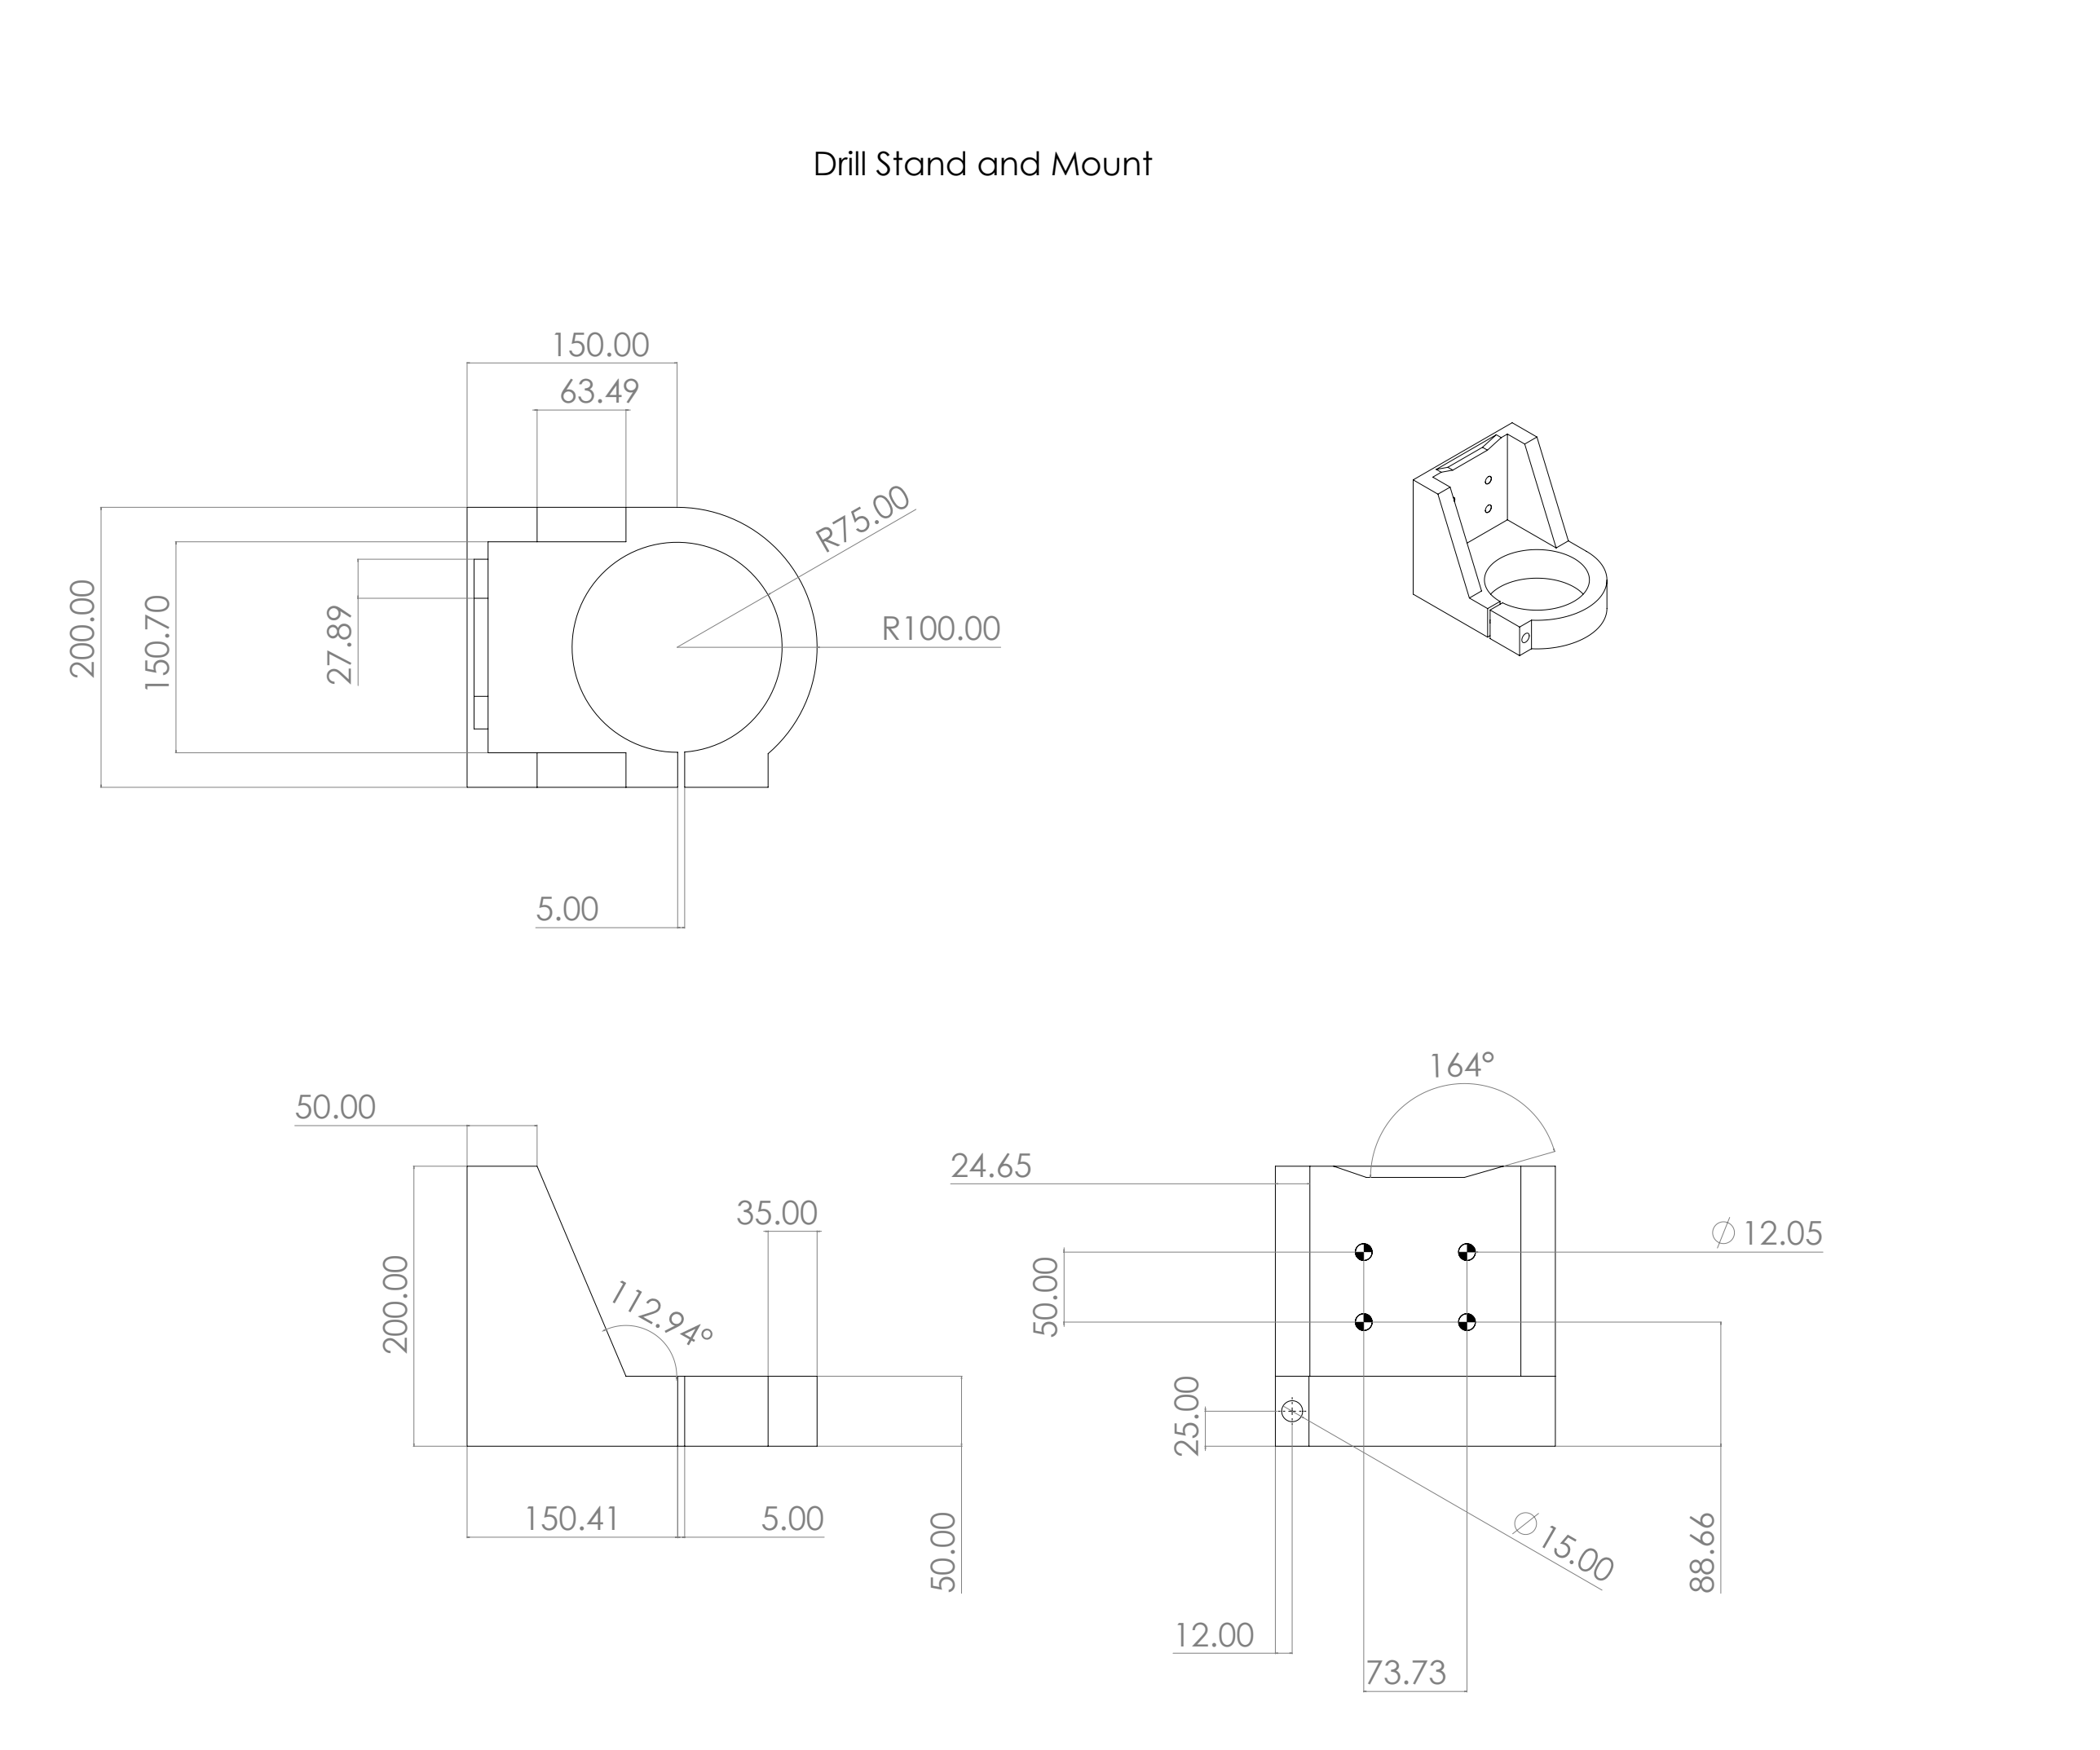
ISO-10303-21;
HEADER;
FILE_DESCRIPTION (('STEP AP214'),
    '1' );
FILE_NAME ('Drill Stand and Mount.step',
    '2026-10-24T00:09:50',
    ( '' ),
    ( '' ),
    'SwSTEP 2.0',
    'SolidWorks 2025',
    '' );
FILE_SCHEMA (( 'AUTOMOTIVE_DESIGN' ));
ENDSEC;

DATA;
#2=CARTESIAN_POINT ( 'NONE',  ( 367.9108539694884144, 44.41075299063183479, 74.99887465166234790 ) ) ;
#16=ORIENTED_EDGE ( 'NONE', *, *, #12011, .T. ) ;
#32=DIRECTION ( 'NONE',  ( 0.000000000000000000, 1.387778780781445182E-16, -1.000000000000000000 ) ) ;
#53=AXIS2_PLACEMENT_3D ( 'NONE', #26136, #19391, #25708 ) ;
#74=DIRECTION ( 'NONE',  ( 1.000000000000000000, -0.000000000000000000, -0.000000000000000000 ) ) ;
#117=VECTOR ( 'NONE', #24571, 1000.000000000000114 ) ;
#119=CIRCLE ( 'NONE', #12970, 75.00000000000002842 ) ;
#146=ORIENTED_EDGE ( 'NONE', *, *, #9436, .T. ) ;
#198=DIRECTION ( 'NONE',  ( 0.000000000000000000, 0.000000000000000000, -1.000000000000000000 ) ) ;
#214=CARTESIAN_POINT ( 'NONE',  ( 232.4999999999996305, 133.0668745871126930, 36.86484227207694886 ) ) ;
#251=CARTESIAN_POINT ( 'NONE',  ( 432.4999999999996589, 44.41075299063184190, 75.99342076785332267 ) ) ;
#260=CARTESIAN_POINT ( 'NONE',  ( 367.9108539694884144, 19.41075299063184900, 87.99671038392668265 ) ) ;
#262=DIRECTION ( 'NONE',  ( -0.000000000000000000, -1.024644424698391667E-16, 1.000000000000000000 ) ) ;
#272=DIRECTION ( 'NONE',  ( 0.000000000000000000, 0.000000000000000000, -1.000000000000000000 ) ) ;
#274=PRODUCT_DEFINITION_CONTEXT ( 'detailed design', #21209, 'design' ) ;
#283=LINE ( 'NONE', #20091, #23680 ) ;
#368=ORIENTED_EDGE ( 'NONE', *, *, #18128, .T. ) ;
#381=CARTESIAN_POINT ( 'NONE',  ( 502.4999999999996021, 44.41075299063184190, 75.35061095560295996 ) ) ;
#396=CARTESIAN_POINT ( 'NONE',  ( 232.4999999999996305, 494.4107529906318632, 75.35061095560301681 ) ) ;
#399=ORIENTED_EDGE ( 'NONE', *, *, #10312, .F. ) ;
#403=CARTESIAN_POINT ( 'NONE',  ( 232.4999999999996305, 494.4107529906318632, -75.35061095560287470 ) ) ;
#431=AXIS2_PLACEMENT_3D ( 'NONE', #7930, #14686, #18707 ) ;
#463=CARTESIAN_POINT ( 'NONE',  ( 267.4999999999996021, 194.4107529906317779, -100.0000000000000000 ) ) ;
#469=LINE ( 'NONE', #26317, #19493 ) ;
#496=DIRECTION ( 'NONE',  ( 0.000000000000000000, -1.000000000000000000, -1.214306433183764966E-16 ) ) ;
#499=DIRECTION ( 'NONE',  ( 0.000000000000000000, 0.000000000000000000, -1.000000000000000000 ) ) ;
#506=VERTEX_POINT ( 'NONE', #21563 ) ;
#545=ORIENTED_EDGE ( 'NONE', *, *, #17891, .F. ) ;
#558=VECTOR ( 'NONE', #22339, 1000.000000000000000 ) ;
#573=CARTESIAN_POINT ( 'NONE',  ( 232.4999999999996305, 44.41075299063184190, 75.35061095560295996 ) ) ;
#598=CIRCLE ( 'NONE', #1034, 7.499999999999992895 ) ;
#629=ORIENTED_EDGE ( 'NONE', *, *, #2343, .F. ) ;
#638=ADVANCED_FACE ( 'NONE', ( #4745 ), #27027, .F. ) ;
#722=ORIENTED_EDGE ( 'NONE', *, *, #6037, .F. ) ;
#743=EDGE_CURVE ( 'NONE', #20178, #23548, #16499, .T. ) ;
#762=ORIENTED_EDGE ( 'NONE', *, *, #3865, .T. ) ;
#776=CARTESIAN_POINT ( 'NONE',  ( 232.4999999999996305, 83.06687458711267880, 42.88984227207694033 ) ) ;
#797=DIRECTION ( 'NONE',  ( 0.000000000000000000, -1.000000000000000000, -1.214306433183764966E-16 ) ) ;
#819=LINE ( 'NONE', #9862, #20338 ) ;
#862=ADVANCED_FACE ( 'NONE', ( #20968 ), #22849, .F. ) ;
#863=VECTOR ( 'NONE', #10211, 1000.000000000000000 ) ;
#913=DIRECTION ( 'NONE',  ( 0.7071067811867438602, 8.659560562352529298E-17, 0.7071067811863512853 ) ) ;
#915=EDGE_LOOP ( 'NONE', ( #27754, #21554, #14846, #21946, #26433, #23940, #8844, #5653, #4028, #10467, #1807, #20190 ) ) ;
#967=ORIENTED_EDGE ( 'NONE', *, *, #14592, .T. ) ;
#1034=AXIS2_PLACEMENT_3D ( 'NONE', #27642, #24944, #3377 ) ;
#1059=AXIS2_PLACEMENT_3D ( 'NONE', #4720, #7463, #22546 ) ;
#1064=EDGE_CURVE ( 'NONE', #27217, #21245, #19801, .T. ) ;
#1075=ORIENTED_EDGE ( 'NONE', *, *, #26791, .T. ) ;
#1077=EDGE_LOOP ( 'NONE', ( #8320, #5448, #967, #19763 ) ) ;
#1096=EDGE_CURVE ( 'NONE', #27590, #27147, #25666, .T. ) ;
#1122=DIRECTION ( 'NONE',  ( -1.000000000000000000, 0.000000000000000000, -9.251858538542972814E-17 ) ) ;
#1154=CIRCLE ( 'NONE', #8503, 7.499999999999992895 ) ;
#1167=ORIENTED_EDGE ( 'NONE', *, *, #1977, .F. ) ;
#1168=AXIS2_PLACEMENT_3D ( 'NONE', #14174, #20345, #22928 ) ;
#1171=CARTESIAN_POINT ( 'NONE',  ( 432.4999999999996589, 19.41075299063184900, 95.49671038392668265 ) ) ;
#1182=EDGE_LOOP ( 'NONE', ( #21901, #2724, #8353, #8644 ) ) ;
#1229=DIRECTION ( 'NONE',  ( 0.000000000000000000, 0.000000000000000000, -1.000000000000000000 ) ) ;
#1251=ORIENTED_EDGE ( 'NONE', *, *, #28136, .T. ) ;
#1273=ORIENTED_EDGE ( 'NONE', *, *, #15927, .F. ) ;
#1283=DIRECTION ( 'NONE',  ( -1.000000000000000000, 0.000000000000000000, -0.000000000000000000 ) ) ;
#1360=EDGE_CURVE ( 'NONE', #5793, #19624, #20048, .T. ) ;
#1366=LINE ( 'NONE', #1775, #8493 ) ;
#1417=ORIENTED_EDGE ( 'NONE', *, *, #15927, .T. ) ;
#1464=MECHANICAL_DESIGN_GEOMETRIC_PRESENTATION_REPRESENTATION('',(#27159),#20745);
#1475=CARTESIAN_POINT ( 'NONE',  ( 282.4999999999996589, 19.41075299063184900, 87.99671038392668265 ) ) ;
#1484=DIRECTION ( 'NONE',  ( 0.000000000000000000, 1.214306433183764720E-16, -1.000000000000000000 ) ) ;
#1522=VECTOR ( 'NONE', #12404, 1000.000000000000000 ) ;
#1529=VECTOR ( 'NONE', #5297, 1000.000000000000000 ) ;
#1542=CARTESIAN_POINT ( 'NONE',  ( 232.4999999999996305, 133.0668745871126930, -30.83984227207694317 ) ) ;
#1550=VECTOR ( 'NONE', #20732, 1000.000000000000000 ) ;
#1571=EDGE_CURVE ( 'NONE', #11251, #16161, #1366, .T. ) ;
#1579=FACE_OUTER_BOUND ( 'NONE', #10470, .T. ) ;
#1613=PLANE ( 'NONE',  #28005 ) ;
#1630=DIRECTION ( 'NONE',  ( 0.000000000000000000, 0.000000000000000000, -1.000000000000000000 ) ) ;
#1644=DIRECTION ( 'NONE',  ( 0.000000000000000000, 0.000000000000000000, -1.000000000000000000 ) ) ;
#1696=ADVANCED_FACE ( 'NONE', ( #27494 ), #7832, .T. ) ;
#1734=FACE_OUTER_BOUND ( 'NONE', #4940, .T. ) ;
#1739=CARTESIAN_POINT ( 'NONE',  ( 232.4749999999995964, 83.06687458711267880, 36.86484227207694175 ) ) ;
#1775=CARTESIAN_POINT ( 'NONE',  ( 232.4999999999996305, 83.06687458711267880, 30.86484227207694886 ) ) ;
#1790=AXIS2_PLACEMENT_3D ( 'NONE', #5010, #4866, #7323 ) ;
#1794=CARTESIAN_POINT ( 'NONE',  ( 222.4999999999996021, 186.4134324495536248, 35.02193266779035952 ) ) ;
#1807=ORIENTED_EDGE ( 'NONE', *, *, #20147, .F. ) ;
#1840=ORIENTED_EDGE ( 'NONE', *, *, #2826, .T. ) ;
#1872=DIRECTION ( 'NONE',  ( 0.000000000000000000, -0.9458112779747414045, 0.3247168404252948615 ) ) ;
#1923=VECTOR ( 'NONE', #18549, 999.9999999999998863 ) ;
#1929=PRODUCT_DEFINITION_FORMATION_WITH_SPECIFIED_SOURCE ( 'ANY', '', #18972, .NOT_KNOWN. ) ;
#1977=EDGE_CURVE ( 'NONE', #23487, #10355, #2919, .T. ) ;
#1990=VECTOR ( 'NONE', #24485, 1000.000000000000000 ) ;
#2018=VERTEX_POINT ( 'NONE', #18010 ) ;
#2020=EDGE_LOOP ( 'NONE', ( #722, #7286, #1075, #6184, #18708, #10466 ) ) ;
#2033=CARTESIAN_POINT ( 'NONE',  ( 232.4999999999996305, 133.0668745871126930, 36.86484227207694886 ) ) ;
#2059=DIRECTION ( 'NONE',  ( 1.000000000000000000, -0.000000000000000000, -0.000000000000000000 ) ) ;
#2080=( NAMED_UNIT ( * ) PLANE_ANGLE_UNIT ( ) SI_UNIT ( $, .RADIAN. ) );
#2084=ORIENTED_EDGE ( 'NONE', *, *, #19529, .F. ) ;
#2085=ADVANCED_FACE ( 'NONE', ( #3611 ), #17365, .F. ) ;
#2130=DIRECTION ( 'NONE',  ( -1.000000000000000000, 0.000000000000000000, -9.251858538542972814E-17 ) ) ;
#2173=DIRECTION ( 'NONE',  ( 1.000000000000000000, -0.000000000000000000, -0.000000000000000000 ) ) ;
#2181=ORIENTED_EDGE ( 'NONE', *, *, #6541, .F. ) ;
#2210=DIRECTION ( 'NONE',  ( 1.000000000000000000, -0.000000000000000000, -0.000000000000000000 ) ) ;
#2216=AXIS2_PLACEMENT_3D ( 'NONE', #2525, #13468, #11754 ) ;
#2227=VERTEX_POINT ( 'NONE', #19949 ) ;
#2269=LINE ( 'NONE', #6873, #2943 ) ;
#2276=LINE ( 'NONE', #21684, #19032 ) ;
#2299=CARTESIAN_POINT ( 'NONE',  ( 232.4999999999996305, 133.0668745871126930, 36.86484227207694886 ) ) ;
#2316=CIRCLE ( 'NONE', #4166, 6.025000000000002132 ) ;
#2320=DIRECTION ( 'NONE',  ( 0.000000000000000000, 0.000000000000000000, 1.000000000000000000 ) ) ;
#2332=ORIENTED_EDGE ( 'NONE', *, *, #13602, .F. ) ;
#2343=EDGE_CURVE ( 'NONE', #9011, #23606, #20659, .T. ) ;
#2431=FACE_OUTER_BOUND ( 'NONE', #26216, .T. ) ;
#2438=CARTESIAN_POINT ( 'NONE',  ( 502.4999999999996021, 494.4107529906318632, -75.35061095560287470 ) ) ;
#2465=ORIENTED_EDGE ( 'NONE', *, *, #10551, .T. ) ;
#2484=DIRECTION ( 'NONE',  ( 0.000000000000000000, 1.272130549049657961E-16, -1.000000000000000000 ) ) ;
#2495=CARTESIAN_POINT ( 'NONE',  ( 232.4999999999996305, 83.06687458711267880, 36.86484227207694175 ) ) ;
#2525=CARTESIAN_POINT ( 'NONE',  ( 367.4999999999996021, -5.589247009368149222, 1.243177022048955014E-14 ) ) ;
#2543=AXIS2_PLACEMENT_3D ( 'NONE', #15014, #19732, #24191 ) ;
#2563=DIRECTION ( 'NONE',  ( 0.000000000000000000, 0.000000000000000000, -1.000000000000000000 ) ) ;
#2642=ORIENTED_EDGE ( 'NONE', *, *, #7765, .T. ) ;
#2649=CARTESIAN_POINT ( 'NONE',  ( 217.4999999999996305, 83.06687458711267880, 42.86484227207692754 ) ) ;
#2657=DIRECTION ( 'NONE',  ( 1.000000000000000000, -0.000000000000000000, -0.000000000000000000 ) ) ;
#2688=EDGE_CURVE ( 'NONE', #12924, #9277, #25082, .T. ) ;
#2697=LINE ( 'NONE', #24831, #15278 ) ;
#2699=AXIS2_PLACEMENT_3D ( 'NONE', #5745, #23135, #25425 ) ;
#2701=EDGE_CURVE ( 'NONE', #26144, #23757, #7603, .T. ) ;
#2717=DIRECTION ( 'NONE',  ( -0.000000000000000000, 0.000000000000000000, 1.000000000000000000 ) ) ;
#2724=ORIENTED_EDGE ( 'NONE', *, *, #25952, .F. ) ;
#2739=DIRECTION ( 'NONE',  ( 0.000000000000000000, 0.000000000000000000, -1.000000000000000000 ) ) ;
#2748=PLANE ( 'NONE',  #7343 ) ;
#2783=EDGE_LOOP ( 'NONE', ( #4645, #20293, #6997, #15217 ) ) ;
#2825=EDGE_LOOP ( 'NONE', ( #22493, #14150, #12355, #13881 ) ) ;
#2826=EDGE_CURVE ( 'NONE', #8811, #11251, #24124, .T. ) ;
#2868=ORIENTED_EDGE ( 'NONE', *, *, #7063, .T. ) ;
#2875=FACE_OUTER_BOUND ( 'NONE', #25974, .T. ) ;
#2876=AXIS2_PLACEMENT_3D ( 'NONE', #26536, #1872, #23869 ) ;
#2919=LINE ( 'NONE', #11703, #13120 ) ;
#2936=EDGE_CURVE ( 'NONE', #7575, #13442, #3014, .T. ) ;
#2943=VECTOR ( 'NONE', #15511, 1000.000000000000000 ) ;
#2944=CARTESIAN_POINT ( 'NONE',  ( 282.4999999999996589, 19.41075299063184900, 95.49671038392668265 ) ) ;
#2946=ORIENTED_EDGE ( 'NONE', *, *, #5275, .T. ) ;
#2947=AXIS2_PLACEMENT_3D ( 'NONE', #24170, #19708, #32 ) ;
#2977=VERTEX_POINT ( 'NONE', #17724 ) ;
#2983=CARTESIAN_POINT ( 'NONE',  ( 367.9108539694884144, 19.41075299063184900, 87.99671038392668265 ) ) ;
#3014=CIRCLE ( 'NONE', #9898, 75.00000000000002842 ) ;
#3017=CARTESIAN_POINT ( 'NONE',  ( 267.4999999999996021, 194.4107529906318064, 75.35061095560300259 ) ) ;
#3036=AXIS2_PLACEMENT_3D ( 'NONE', #20911, #5961, #12167 ) ;
#3045=DIRECTION ( 'NONE',  ( 0.000000000000000000, -0.000000000000000000, -1.000000000000000000 ) ) ;
#3065=CARTESIAN_POINT ( 'NONE',  ( 217.4999999999996305, 194.4107529906318064, -100.0000000000000000 ) ) ;
#3082=EDGE_LOOP ( 'NONE', ( #22866, #18073, #13925, #14229, #8531, #24826, #24828, #23547, #2946, #19715, #21670 ) ) ;
#3115=DIRECTION ( 'NONE',  ( 0.000000000000000000, 0.000000000000000000, 1.000000000000000000 ) ) ;
#3129=CARTESIAN_POINT ( 'NONE',  ( 330.9869376377542949, 44.41075299063183479, 288.0938197134494203 ) ) ;
#3165=DIRECTION ( 'NONE',  ( -1.000000000000000000, 0.000000000000000000, -0.000000000000000000 ) ) ;
#3199=ORIENTED_EDGE ( 'NONE', *, *, #28136, .F. ) ;
#3201=FACE_OUTER_BOUND ( 'NONE', #15790, .T. ) ;
#3215=CARTESIAN_POINT ( 'NONE',  ( 367.4999999999996021, 44.41075299063184900, 1.850330238640837654E-14 ) ) ;
#3216=ORIENTED_EDGE ( 'NONE', *, *, #8413, .T. ) ;
#3262=AXIS2_PLACEMENT_3D ( 'NONE', #21260, #14812, #17096 ) ;
#3268=DIRECTION ( 'NONE',  ( -0.000000000000000000, -0.000000000000000000, -1.000000000000000000 ) ) ;
#3274=ADVANCED_FACE ( 'NONE', ( #2875 ), #11668, .F. ) ;
#3284=AXIS2_PLACEMENT_3D ( 'NONE', #3500, #3782, #21026 ) ;
#3318=LINE ( 'NONE', #16414, #20270 ) ;
#3357=ORIENTED_EDGE ( 'NONE', *, *, #2688, .F. ) ;
#3363=ORIENTED_EDGE ( 'NONE', *, *, #15631, .T. ) ;
#3377=DIRECTION ( 'NONE',  ( 0.000000000000000000, 0.000000000000000000, -1.000000000000000000 ) ) ;
#3401=EDGE_CURVE ( 'NONE', #25274, #17486, #27497, .T. ) ;
#3414=LINE ( 'NONE', #3129, #3708 ) ;
#3427=ADVANCED_FACE ( 'NONE', ( #24692 ), #13792, .T. ) ;
#3443=PLANE ( 'NONE',  #2699 ) ;
#3473=CARTESIAN_POINT ( 'NONE',  ( 367.4999999999996021, -5.589247009368158103, 75.00000000000004263 ) ) ;
#3476=DIRECTION ( 'NONE',  ( -0.9209112846414913012, -0.3897722486529259789, 0.000000000000000000 ) ) ;
#3500=CARTESIAN_POINT ( 'NONE',  ( 217.4999999999996305, 44.41075299063186321, -100.0000000000000142 ) ) ;
#3549=EDGE_CURVE ( 'NONE', #18668, #22380, #28356, .T. ) ;
#3571=ORIENTED_EDGE ( 'NONE', *, *, #1096, .T. ) ;
#3611=FACE_OUTER_BOUND ( 'NONE', #25231, .T. ) ;
#3681=ORIENTED_EDGE ( 'NONE', *, *, #22426, .T. ) ;
#3708=VECTOR ( 'NONE', #3268, 1000.000000000000000 ) ;
#3782=DIRECTION ( 'NONE',  ( 0.000000000000000000, 1.214306433183764966E-16, -1.000000000000000000 ) ) ;
#3783=FACE_OUTER_BOUND ( 'NONE', #18224, .T. ) ;
#3787=DIRECTION ( 'NONE',  ( 0.000000000000000000, 0.000000000000000000, -1.000000000000000000 ) ) ;
#3799=CIRCLE ( 'NONE', #22158, 7.499999999999992895 ) ;
#3813=DIRECTION ( 'NONE',  ( 1.000000000000000000, -0.000000000000000000, -0.000000000000000000 ) ) ;
#3832=EDGE_CURVE ( 'NONE', #26471, #23612, #24621, .T. ) ;
#3849=ORIENTED_EDGE ( 'NONE', *, *, #22423, .T. ) ;
#3865=EDGE_CURVE ( 'NONE', #23487, #2018, #24718, .T. ) ;
#3909=FACE_OUTER_BOUND ( 'NONE', #1077, .T. ) ;
#3923=PLANE ( 'NONE',  #3284 ) ;
#3929=ORIENTED_EDGE ( 'NONE', *, *, #9136, .F. ) ;
#3942=ORIENTED_EDGE ( 'NONE', *, *, #20538, .T. ) ;
#3951=FACE_OUTER_BOUND ( 'NONE', #15568, .T. ) ;
#4026=AXIS2_PLACEMENT_3D ( 'NONE', #8368, #19568, #8512 ) ;
#4028=ORIENTED_EDGE ( 'NONE', *, *, #12389, .T. ) ;
#4056=CARTESIAN_POINT ( 'NONE',  ( 502.4999999999996021, 44.41075299063185611, -75.35061095560293154 ) ) ;
#4075=CARTESIAN_POINT ( 'NONE',  ( 232.4999999999996305, 133.0668745871126930, 36.86484227207694886 ) ) ;
#4078=DIRECTION ( 'NONE',  ( -0.000000000000000000, 0.2756732917354685064, -0.9612513907525602752 ) ) ;
#4084=CARTESIAN_POINT ( 'NONE',  ( 367.4999999999996021, 44.41075299063184900, 1.850330238640837654E-14 ) ) ;
#4105=EDGE_LOOP ( 'NONE', ( #25695, #5890, #24042, #26859 ) ) ;
#4130=ORIENTED_EDGE ( 'NONE', *, *, #8999, .F. ) ;
#4166=AXIS2_PLACEMENT_3D ( 'NONE', #13541, #19846, #5042 ) ;
#4176=VERTEX_POINT ( 'NONE', #18404 ) ;
#4263=DIRECTION ( 'NONE',  ( -0.000000000000000000, -0.000000000000000000, -1.000000000000000000 ) ) ;
#4266=CARTESIAN_POINT ( 'NONE',  ( 372.9108539694884144, -280.0000000000000568, 167.7200181511720132 ) ) ;
#4281=LINE ( 'NONE', #403, #10536 ) ;
#4286=ORIENTED_EDGE ( 'NONE', *, *, #7759, .F. ) ;
#4293=ADVANCED_FACE ( 'NONE', ( #21255, #14245, #12511, #7902, #16673 ), #3443, .T. ) ;
#4306=ORIENTED_EDGE ( 'NONE', *, *, #13602, .T. ) ;
#4325=FACE_OUTER_BOUND ( 'NONE', #11853, .T. ) ;
#4328=DIRECTION ( 'NONE',  ( 1.000000000000000000, -0.000000000000000000, -0.000000000000000000 ) ) ;
#4332=DIRECTION ( 'NONE',  ( 0.000000000000000000, 0.000000000000000000, -1.000000000000000000 ) ) ;
#4398=CARTESIAN_POINT ( 'NONE',  ( 217.4999999999996305, 133.0668745871126930, 42.86484227207692044 ) ) ;
#4430=DIRECTION ( 'NONE',  ( 0.000000000000000000, -1.000000000000000000, -1.214306433183764966E-16 ) ) ;
#4444=VECTOR ( 'NONE', #14125, 1000.000000000000000 ) ;
#4449=EDGE_LOOP ( 'NONE', ( #6153, #27694, #15526, #26157 ) ) ;
#4534=ADVANCED_FACE ( 'NONE', ( #11056 ), #19809, .F. ) ;
#4555=CARTESIAN_POINT ( 'NONE',  ( 367.9108539694884144, 44.41075299063183479, 167.7200181511720416 ) ) ;
#4563=CARTESIAN_POINT ( 'NONE',  ( 232.4749999999995964, 133.0668745871126930, 30.86484227207697018 ) ) ;
#4566=UNCERTAINTY_MEASURE_WITH_UNIT (LENGTH_MEASURE( 1.000000000000000082E-05 ), #22156, 'distance_accuracy_value', 'NONE');
#4567=CARTESIAN_POINT ( 'NONE',  ( 232.4999999999996305, 83.06687458711267880, 36.86484227207694175 ) ) ;
#4633=DIRECTION ( 'NONE',  ( 1.000000000000000000, 0.000000000000000000, 0.000000000000000000 ) ) ;
#4636=DIRECTION ( 'NONE',  ( 0.000000000000000000, 0.2756732917354685064, -0.9612513907525602752 ) ) ;
#4645=ORIENTED_EDGE ( 'NONE', *, *, #18540, .F. ) ;
#4675=CIRCLE ( 'NONE', #8361, 5.999999999999991118 ) ;
#4702=EDGE_CURVE ( 'NONE', #5949, #12519, #23528, .T. ) ;
#4708=ADVANCED_FACE ( 'NONE', ( #18520 ), #16434, .F. ) ;
#4720=CARTESIAN_POINT ( 'NONE',  ( 232.4999999999996305, 494.4107529906318632, 75.35061095560301681 ) ) ;
#4736=EDGE_CURVE ( 'NONE', #9830, #15470, #16371, .T. ) ;
#4745=FACE_OUTER_BOUND ( 'NONE', #22806, .T. ) ;
#4767=ORIENTED_EDGE ( 'NONE', *, *, #2701, .F. ) ;
#4788=DIRECTION ( 'NONE',  ( 0.000000000000000000, 1.214306433183764966E-16, -1.000000000000000000 ) ) ;
#4803=CARTESIAN_POINT ( 'NONE',  ( 222.4999999999996021, 186.4134324495536248, 35.02193266779035952 ) ) ;
#4810=ORIENTED_EDGE ( 'NONE', *, *, #10551, .F. ) ;
#4833=LINE ( 'NONE', #13913, #18573 ) ;
#4858=ADVANCED_FACE ( 'NONE', ( #6281, #19775 ), #15055, .F. ) ;
#4866=DIRECTION ( 'NONE',  ( 1.000000000000000000, -0.000000000000000000, -0.000000000000000000 ) ) ;
#4874=EDGE_CURVE ( 'NONE', #25738, #8109, #28102, .T. ) ;
#4940=EDGE_LOOP ( 'NONE', ( #13871, #12734, #13301, #11446 ) ) ;
#4980=EDGE_CURVE ( 'NONE', #22380, #7575, #6342, .T. ) ;
#4981=CARTESIAN_POINT ( 'NONE',  ( 217.4999999999996305, 194.4107529906318064, 100.0000000000000284 ) ) ;
#5010=CARTESIAN_POINT ( 'NONE',  ( 232.4999999999996305, 83.06687458711267880, -36.86484227207694175 ) ) ;
#5042=DIRECTION ( 'NONE',  ( 0.000000000000000000, 0.000000000000000000, -1.000000000000000000 ) ) ;
#5044=CARTESIAN_POINT ( 'NONE',  ( 217.4999999999996305, 83.06687458711267880, -36.86484227207694175 ) ) ;
#5045=ORIENTED_EDGE ( 'NONE', *, *, #6467, .F. ) ;
#5047=CARTESIAN_POINT ( 'NONE',  ( 367.4999999999996021, 44.41075299063184900, 1.850330238640837654E-14 ) ) ;
#5057=ADVANCED_BREP_SHAPE_REPRESENTATION ( '', ( #8800, #10637 ), #20272 ) ;
#5120=ORIENTED_EDGE ( 'NONE', *, *, #13622, .F. ) ;
#5156=AXIS2_PLACEMENT_3D ( 'NONE', #7372, #12115, #3045 ) ;
#5241=DIRECTION ( 'NONE',  ( 0.000000000000000000, 1.000000000000000000, 1.214306433183764966E-16 ) ) ;
#5261=AXIS2_PLACEMENT_3D ( 'NONE', #17632, #28252, #25824 ) ;
#5275=EDGE_CURVE ( 'NONE', #12260, #15470, #5914, .T. ) ;
#5297=DIRECTION ( 'NONE',  ( -1.000000000000000000, 0.000000000000000000, 0.000000000000000000 ) ) ;
#5306=ORIENTED_EDGE ( 'NONE', *, *, #17384, .T. ) ;
#5316=CARTESIAN_POINT ( 'NONE',  ( 232.4999999999996305, 83.06687458711267880, -36.86484227207694175 ) ) ;
#5339=CIRCLE ( 'NONE', #3036, 75.00000000000002842 ) ;
#5419=CARTESIAN_POINT ( 'NONE',  ( 282.4999999999996589, 19.41075299063184900, 80.49671038392669686 ) ) ;
#5448=ORIENTED_EDGE ( 'NONE', *, *, #15059, .F. ) ;
#5521=DIRECTION ( 'NONE',  ( 1.000000000000000000, -0.000000000000000000, -0.000000000000000000 ) ) ;
#5559=EDGE_CURVE ( 'NONE', #17744, #5793, #16676, .T. ) ;
#5587=CARTESIAN_POINT ( 'NONE',  ( 232.4999999999996305, 186.4134324495536248, -35.02193266779035952 ) ) ;
#5610=CARTESIAN_POINT ( 'NONE',  ( 222.4999999999996021, 0.000000000000000000, 0.000000000000000000 ) ) ;
#5614=DIRECTION ( 'NONE',  ( 1.000000000000000000, 0.000000000000000000, 0.000000000000000000 ) ) ;
#5627=AXIS2_PLACEMENT_3D ( 'NONE', #21043, #25363, #1229 ) ;
#5647=AXIS2_PLACEMENT_3D ( 'NONE', #2495, #2210, #11285 ) ;
#5653=ORIENTED_EDGE ( 'NONE', *, *, #14358, .F. ) ;
#5745=CARTESIAN_POINT ( 'NONE',  ( 217.4999999999996305, 44.41075299063183479, 100.0000000000000142 ) ) ;
#5767=ORIENTED_EDGE ( 'NONE', *, *, #6544, .F. ) ;
#5769=LINE ( 'NONE', #10231, #12506 ) ;
#5791=ORIENTED_EDGE ( 'NONE', *, *, #28135, .T. ) ;
#5793=VERTEX_POINT ( 'NONE', #573 ) ;
#5808=VERTEX_POINT ( 'NONE', #7467 ) ;
#5810=ORIENTED_EDGE ( 'NONE', *, *, #7765, .F. ) ;
#5834=DIRECTION ( 'NONE',  ( 1.000000000000000000, 0.000000000000000000, 0.000000000000000000 ) ) ;
#5859=ADVANCED_FACE ( 'NONE', ( #24704 ), #17949, .F. ) ;
#5890=ORIENTED_EDGE ( 'NONE', *, *, #10649, .T. ) ;
#5895=ORIENTED_EDGE ( 'NONE', *, *, #11648, .F. ) ;
#5897=ORIENTED_EDGE ( 'NONE', *, *, #21978, .T. ) ;
#5902=EDGE_LOOP ( 'NONE', ( #11688, #4767 ) ) ;
#5910=ORIENTED_EDGE ( 'NONE', *, *, #2936, .T. ) ;
#5911=FACE_OUTER_BOUND ( 'NONE', #4105, .T. ) ;
#5913=DIRECTION ( 'NONE',  ( 0.7071067811865474617, 8.659560562354932858E-17, 0.7071067811865474617 ) ) ;
#5914=CIRCLE ( 'NONE', #22432, 100.0000000000000284 ) ;
#5920=AXIS2_PLACEMENT_3D ( 'NONE', #2299, #8923, #15973 ) ;
#5925=CARTESIAN_POINT ( 'NONE',  ( 232.4999999999996305, 83.06687458711267880, 42.88984227207694033 ) ) ;
#5930=EDGE_LOOP ( 'NONE', ( #1167, #21949, #23539, #4306 ) ) ;
#5938=DIRECTION ( 'NONE',  ( 0.000000000000000000, -1.000000000000000000, -1.214306433183764966E-16 ) ) ;
#5946=CYLINDRICAL_SURFACE ( 'NONE', #20961, 7.499999999999992895 ) ;
#5949=VERTEX_POINT ( 'NONE', #8308 ) ;
#5957=AXIS2_PLACEMENT_3D ( 'NONE', #19610, #25787, #25928 ) ;
#5961=DIRECTION ( 'NONE',  ( 0.000000000000000000, -1.000000000000000000, -1.214306433183764966E-16 ) ) ;
#5981=APPLICATION_CONTEXT ( 'automotive_design' ) ;
#6024=CARTESIAN_POINT ( 'NONE',  ( 222.4999999999996021, 194.4107529906318064, -62.90796922943941638 ) ) ;
#6030=CARTESIAN_POINT ( 'NONE',  ( 232.4999999999996305, 44.41075299063184190, 75.35061095560295996 ) ) ;
#6037=EDGE_CURVE ( 'NONE', #9011, #27217, #14634, .T. ) ;
#6040=ORIENTED_EDGE ( 'NONE', *, *, #12231, .T. ) ;
#6047=EDGE_LOOP ( 'NONE', ( #16873, #9356, #10053, #17070 ) ) ;
#6050=AXIS2_PLACEMENT_3D ( 'NONE', #1475, #23178, #14851 ) ;
#6054=CARTESIAN_POINT ( 'NONE',  ( 232.4749999999995964, 133.0668745871126930, 42.86484227207692044 ) ) ;
#6091=CARTESIAN_POINT ( 'NONE',  ( 222.4999999999996021, 186.4134324495536248, -35.02193266779035952 ) ) ;
#6102=ORIENTED_EDGE ( 'NONE', *, *, #5275, .F. ) ;
#6117=CARTESIAN_POINT ( 'NONE',  ( 372.9108539694884144, 44.41075299063183479, 74.80456309157131045 ) ) ;
#6118=EDGE_LOOP ( 'NONE', ( #7668, #22373, #5910, #21610 ) ) ;
#6145=FACE_OUTER_BOUND ( 'NONE', #19193, .T. ) ;
#6153=ORIENTED_EDGE ( 'NONE', *, *, #28236, .F. ) ;
#6184=ORIENTED_EDGE ( 'NONE', *, *, #14358, .T. ) ;
#6191=VECTOR ( 'NONE', #14804, 1000.000000000000000 ) ;
#6229=ORIENTED_EDGE ( 'NONE', *, *, #14714, .F. ) ;
#6280=CARTESIAN_POINT ( 'NONE',  ( 367.9108539694884144, -5.589247009368157215, 74.99887465166234790 ) ) ;
#6281=FACE_BOUND ( 'NONE', #16596, .T. ) ;
#6290=DIRECTION ( 'NONE',  ( 0.000000000000000000, -1.000000000000000000, -1.214306433183764966E-16 ) ) ;
#6294=EDGE_CURVE ( 'NONE', #8492, #5793, #20064, .T. ) ;
#6322=VECTOR ( 'NONE', #27537, 1000.000000000000000 ) ;
#6342=CIRCLE ( 'NONE', #2216, 75.00000000000002842 ) ;
#6346=CARTESIAN_POINT ( 'NONE',  ( 367.9108539694884144, -280.0000000000000568, 167.7200181511720132 ) ) ;
#6443=ORIENTED_EDGE ( 'NONE', *, *, #6541, .T. ) ;
#6467=EDGE_CURVE ( 'NONE', #9950, #15333, #14681, .T. ) ;
#6481=ORIENTED_EDGE ( 'NONE', *, *, #27821, .F. ) ;
#6492=LINE ( 'NONE', #14988, #17920 ) ;
#6541=EDGE_CURVE ( 'NONE', #2227, #12260, #17591, .T. ) ;
#6544=EDGE_CURVE ( 'NONE', #9950, #20572, #21908, .T. ) ;
#6591=UNCERTAINTY_MEASURE_WITH_UNIT (LENGTH_MEASURE( 1.000000000000000082E-05 ), #17884, 'distance_accuracy_value', 'NONE');
#6635=CARTESIAN_POINT ( 'NONE',  ( 217.4999999999996305, 194.4107529906318064, -75.35061095560291733 ) ) ;
#6642=DIRECTION ( 'NONE',  ( -0.000000000000000000, -0.000000000000000000, -1.000000000000000000 ) ) ;
#6652=CARTESIAN_POINT ( 'NONE',  ( 232.4999999999996305, 133.0668745871126930, -30.83984227207694317 ) ) ;
#6673=CARTESIAN_POINT ( 'NONE',  ( 222.4999999999996021, 186.4134324495536248, -35.02193266779035952 ) ) ;
#6686=ORIENTED_EDGE ( 'NONE', *, *, #15833, .F. ) ;
#6706=ORIENTED_EDGE ( 'NONE', *, *, #11340, .F. ) ;
#6733=DIRECTION ( 'NONE',  ( 1.000000000000000000, 0.000000000000000000, 0.000000000000000000 ) ) ;
#6738=DIRECTION ( 'NONE',  ( 0.000000000000000000, 1.000000000000000000, 1.214306433183764966E-16 ) ) ;
#6742=CIRCLE ( 'NONE', #20511, 5.999999999999977796 ) ;
#6777=DIRECTION ( 'NONE',  ( 1.000000000000000000, 0.000000000000000000, 0.000000000000000000 ) ) ;
#6803=DIRECTION ( 'NONE',  ( 0.000000000000000000, 1.387778780781445182E-16, -1.000000000000000000 ) ) ;
#6873=CARTESIAN_POINT ( 'NONE',  ( 232.4999999999996305, 194.4107529906318064, 288.0938197134494203 ) ) ;
#6888=EDGE_LOOP ( 'NONE', ( #24221, #12671, #19443, #20155 ) ) ;
#6894=EDGE_LOOP ( 'NONE', ( #10162, #3199, #25412, #6040 ) ) ;
#6941=EDGE_CURVE ( 'NONE', #13442, #25647, #10676, .T. ) ;
#6949=DIRECTION ( 'NONE',  ( 1.000000000000000000, 0.000000000000000000, 0.000000000000000000 ) ) ;
#6959=LINE ( 'NONE', #4803, #558 ) ;
#6969=EDGE_LOOP ( 'NONE', ( #17569, #7993 ) ) ;
#6997=ORIENTED_EDGE ( 'NONE', *, *, #22454, .T. ) ;
#7026=VECTOR ( 'NONE', #15775, 1000.000000000000000 ) ;
#7046=CARTESIAN_POINT ( 'NONE',  ( 232.4999999999996305, 83.06687458711267880, -30.83984227207693607 ) ) ;
#7063=EDGE_CURVE ( 'NONE', #17486, #25274, #22035, .T. ) ;
#7076=EDGE_CURVE ( 'NONE', #26636, #22380, #12512, .T. ) ;
#7149=DIRECTION ( 'NONE',  ( -1.000000000000000000, 0.000000000000000000, -0.000000000000000000 ) ) ;
#7154=VERTEX_POINT ( 'NONE', #10481 ) ;
#7190=VECTOR ( 'NONE', #19587, 1000.000000000000114 ) ;
#7224=CARTESIAN_POINT ( 'NONE',  ( 232.4999999999996305, 133.0668745871126930, -42.88984227207694744 ) ) ;
#7237=DIRECTION ( 'NONE',  ( 1.000000000000000000, -0.000000000000000000, -0.000000000000000000 ) ) ;
#7250=DIRECTION ( 'NONE',  ( 1.000000000000000000, -0.000000000000000000, -0.000000000000000000 ) ) ;
#7276=ADVANCED_FACE ( 'NONE', ( #15205 ), #15490, .F. ) ;
#7277=CARTESIAN_POINT ( 'NONE',  ( 232.4999999999996305, 44.41075299063185611, -75.35061095560293154 ) ) ;
#7286=ORIENTED_EDGE ( 'NONE', *, *, #2343, .T. ) ;
#7290=AXIS2_PLACEMENT_3D ( 'NONE', #16778, #7870, #22824 ) ;
#7295=ORIENTED_EDGE ( 'NONE', *, *, #8807, .T. ) ;
#7323=DIRECTION ( 'NONE',  ( 0.000000000000000000, 0.000000000000000000, -1.000000000000000000 ) ) ;
#7343=AXIS2_PLACEMENT_3D ( 'NONE', #22586, #15989, #7502 ) ;
#7372=CARTESIAN_POINT ( 'NONE',  ( 217.4999999999996305, 194.4107529906318064, 288.0938197134494203 ) ) ;
#7405=CIRCLE ( 'NONE', #24832, 6.025000000000002132 ) ;
#7410=DIRECTION ( 'NONE',  ( 0.000000000000000000, 0.000000000000000000, -1.000000000000000000 ) ) ;
#7435=CARTESIAN_POINT ( 'NONE',  ( 232.4999999999996305, 194.4107529906318064, 75.35061095560297417 ) ) ;
#7440=EDGE_CURVE ( 'NONE', #2977, #7154, #20209, .T. ) ;
#7463=DIRECTION ( 'NONE',  ( 1.000000000000000000, 0.000000000000000000, 0.000000000000000000 ) ) ;
#7467=CARTESIAN_POINT ( 'NONE',  ( 217.4999999999996305, -5.589247009368136787, -100.0000000000000142 ) ) ;
#7480=VERTEX_POINT ( 'NONE', #5925 ) ;
#7484=VECTOR ( 'NONE', #18367, 1000.000000000000000 ) ;
#7488=CARTESIAN_POINT ( 'NONE',  ( 232.4999999999996305, 83.06687458711267880, 36.86484227207694175 ) ) ;
#7496=CARTESIAN_POINT ( 'NONE',  ( 222.4999999999996021, 186.4134324495536248, -35.02193266779035952 ) ) ;
#7502=DIRECTION ( 'NONE',  ( 0.3897722486529259234, -0.9209112846414911902, 0.000000000000000000 ) ) ;
#7504=DIRECTION ( 'NONE',  ( 0.000000000000000000, -1.000000000000000000, -1.214306433183764966E-16 ) ) ;
#7516=CARTESIAN_POINT ( 'NONE',  ( 222.4999999999996021, 194.4107529906318064, -62.90796922943941638 ) ) ;
#7537=CARTESIAN_POINT ( 'NONE',  ( 222.4999999999996021, 194.4107529906318064, 58.31593845887894645 ) ) ;
#7543=LINE ( 'NONE', #25476, #19037 ) ;
#7553=ORIENTED_EDGE ( 'NONE', *, *, #1360, .T. ) ;
#7559=ADVANCED_FACE ( 'NONE', ( #23735 ), #19760, .F. ) ;
#7575=VERTEX_POINT ( 'NONE', #25740 ) ;
#7602=DIRECTION ( 'NONE',  ( 0.000000000000000000, 0.000000000000000000, -1.000000000000000000 ) ) ;
#7603=CIRCLE ( 'NONE', #1168, 6.025000000000002132 ) ;
#7619=AXIS2_PLACEMENT_3D ( 'NONE', #27597, #3476, #23984 ) ;
#7623=DIRECTION ( 'NONE',  ( -9.251858538542974046E-17, -1.214306433183764966E-16, 1.000000000000000000 ) ) ;
#7624=EDGE_CURVE ( 'NONE', #12356, #16763, #6492, .T. ) ;
#7632=ADVANCED_FACE ( 'NONE', ( #19284, #19571 ), #1613, .F. ) ;
#7641=EDGE_CURVE ( 'NONE', #23548, #20178, #2316, .T. ) ;
#7649=DIRECTION ( 'NONE',  ( 0.7071067811867438602, 0.000000000000000000, -0.7071067811863512853 ) ) ;
#7651=ORIENTED_EDGE ( 'NONE', *, *, #8934, .T. ) ;
#7668=ORIENTED_EDGE ( 'NONE', *, *, #8934, .F. ) ;
#7669=CARTESIAN_POINT ( 'NONE',  ( 432.4999999999996589, -5.589247009368158103, 75.99342076785332267 ) ) ;
#7685=CLOSED_SHELL ( 'NONE', ( #27662, #5859, #10923, #13213, #638, #25140, #12744, #862, #18950, #19519, #7276, #21054, #26875, #12538, #12366, #2085, #16790, #21383, #15295, #4293, #3427, #10099, #7950, #11235, #9891, #10487, #18643, #7632, #4858, #26174, #23715, #1696, #14081, #13988, #21540, #15788, #18376, #21415, #23268, #16251, #4534, #4708, #3274, #7559 ) ) ;
#7720=AXIS2_PLACEMENT_3D ( 'NONE', #4084, #10706, #6803 ) ;
#7759=EDGE_CURVE ( 'NONE', #27147, #23757, #27294, .T. ) ;
#7765=EDGE_CURVE ( 'NONE', #8109, #8669, #20694, .T. ) ;
#7775=DIRECTION ( 'NONE',  ( 0.000000000000000000, 0.000000000000000000, -1.000000000000000000 ) ) ;
#7812=AXIS2_PLACEMENT_3D ( 'NONE', #24129, #25985, #17652 ) ;
#7825=FACE_OUTER_BOUND ( 'NONE', #5930, .T. ) ;
#7827=VECTOR ( 'NONE', #4078, 1000.000000000000000 ) ;
#7832=PLANE ( 'NONE',  #11266 ) ;
#7865=EDGE_CURVE ( 'NONE', #23614, #17607, #12009, .T. ) ;
#7870=DIRECTION ( 'NONE',  ( 0.000000000000000000, -1.000000000000000000, -1.214306433183764966E-16 ) ) ;
#7885=ORIENTED_EDGE ( 'NONE', *, *, #6941, .T. ) ;
#7893=ORIENTED_EDGE ( 'NONE', *, *, #21439, .T. ) ;
#7902=FACE_BOUND ( 'NONE', #21379, .T. ) ;
#7908=CARTESIAN_POINT ( 'NONE',  ( 232.4999999999996305, 133.0668745871126930, 30.83984227207694317 ) ) ;
#7930=CARTESIAN_POINT ( 'NONE',  ( 232.4999999999996305, 83.06687458711267880, -36.86484227207694175 ) ) ;
#7950=ADVANCED_FACE ( 'NONE', ( #27995 ), #16818, .T. ) ;
#7952=ORIENTED_EDGE ( 'NONE', *, *, #28236, .T. ) ;
#7993=ORIENTED_EDGE ( 'NONE', *, *, #6467, .T. ) ;
#7996=CARTESIAN_POINT ( 'NONE',  ( 217.4999999999996305, 194.4107529906318064, 75.35061095560300259 ) ) ;
#8019=VERTEX_POINT ( 'NONE', #2 ) ;
#8036=CARTESIAN_POINT ( 'NONE',  ( 367.4999999999996021, 44.41075299063183479, 100.0000000000000284 ) ) ;
#8084=EDGE_LOOP ( 'NONE', ( #2332, #11399 ) ) ;
#8090=LINE ( 'NONE', #21435, #26330 ) ;
#8104=CARTESIAN_POINT ( 'NONE',  ( 232.4999999999996305, 133.0668745871126930, 36.86484227207694886 ) ) ;
#8109=VERTEX_POINT ( 'NONE', #21970 ) ;
#8145=EDGE_CURVE ( 'NONE', #25647, #8109, #11354, .T. ) ;
#8187=AXIS2_PLACEMENT_3D ( 'NONE', #5610, #20975, #14523 ) ;
#8196=VECTOR ( 'NONE', #11564, 1000.000000000000000 ) ;
#8223=AXIS2_PLACEMENT_3D ( 'NONE', #22103, #17647, #272 ) ;
#8249=ORIENTED_EDGE ( 'NONE', *, *, #16395, .F. ) ;
#8284=CARTESIAN_POINT ( 'NONE',  ( 432.4999999999996589, 44.41075299063184190, 100.0000000000000426 ) ) ;
#8308=CARTESIAN_POINT ( 'NONE',  ( 222.4999999999996021, 194.4107529906318064, -62.90796922943941638 ) ) ;
#8320=ORIENTED_EDGE ( 'NONE', *, *, #7076, .F. ) ;
#8353=ORIENTED_EDGE ( 'NONE', *, *, #7759, .T. ) ;
#8361=AXIS2_PLACEMENT_3D ( 'NONE', #13102, #28151, #19828 ) ;
#8368=CARTESIAN_POINT ( 'NONE',  ( 232.4749999999995964, 83.06687458711267880, 36.86484227207694175 ) ) ;
#8386=AXIS2_PLACEMENT_3D ( 'NONE', #22410, #9345, #10679 ) ;
#8413=EDGE_CURVE ( 'NONE', #14199, #12077, #26383, .T. ) ;
#8417=CARTESIAN_POINT ( 'NONE',  ( 232.4999999999996305, 133.0668745871126930, -36.86484227207694886 ) ) ;
#8446=CIRCLE ( 'NONE', #17152, 7.499999999999992895 ) ;
#8492=VERTEX_POINT ( 'NONE', #7435 ) ;
#8493=VECTOR ( 'NONE', #21460, 1000.000000000000000 ) ;
#8503=AXIS2_PLACEMENT_3D ( 'NONE', #26448, #6777, #20285 ) ;
#8504=CARTESIAN_POINT ( 'NONE',  ( 232.4999999999996305, 133.0668745871126930, 42.88984227207694744 ) ) ;
#8510=LINE ( 'NONE', #28304, #13371 ) ;
#8512=DIRECTION ( 'NONE',  ( 0.000000000000000000, 0.000000000000000000, -1.000000000000000000 ) ) ;
#8531=ORIENTED_EDGE ( 'NONE', *, *, #21543, .F. ) ;
#8544=VECTOR ( 'NONE', #15052, 1000.000000000000000 ) ;
#8554=DIRECTION ( 'NONE',  ( 0.000000000000000000, -1.000000000000000000, -1.214306433183764966E-16 ) ) ;
#8644=ORIENTED_EDGE ( 'NONE', *, *, #18445, .T. ) ;
#8655=CARTESIAN_POINT ( 'NONE',  ( 232.4999999999996305, 83.06687458711267880, -36.86484227207694175 ) ) ;
#8667=VECTOR ( 'NONE', #22291, 1000.000000000000000 ) ;
#8669=VERTEX_POINT ( 'NONE', #6117 ) ;
#8721=LINE ( 'NONE', #9005, #20015 ) ;
#8770=ORIENTED_EDGE ( 'NONE', *, *, #4874, .T. ) ;
#8782=AXIS2_PLACEMENT_3D ( 'NONE', #26095, #21226, #13054 ) ;
#8783=CYLINDRICAL_SURFACE ( 'NONE', #24513, 7.499999999999992895 ) ;
#8785=VECTOR ( 'NONE', #15600, 1000.000000000000000 ) ;
#8800=MANIFOLD_SOLID_BREP ( '\X2\00d8\X0\12.0mm Dowel Hole2[2]', #7685 ) ;
#8807=EDGE_CURVE ( 'NONE', #12519, #26013, #6959, .T. ) ;
#8811=VERTEX_POINT ( 'NONE', #2649 ) ;
#8844=ORIENTED_EDGE ( 'NONE', *, *, #14697, .F. ) ;
#8848=VECTOR ( 'NONE', #2717, 1000.000000000000000 ) ;
#8850=ORIENTED_EDGE ( 'NONE', *, *, #15590, .T. ) ;
#8923=DIRECTION ( 'NONE',  ( 1.000000000000000000, -0.000000000000000000, -0.000000000000000000 ) ) ;
#8934=EDGE_CURVE ( 'NONE', #23123, #8669, #119, .T. ) ;
#8953=CARTESIAN_POINT ( 'NONE',  ( 217.4999999999996305, -5.589247009368160768, 100.0000000000000142 ) ) ;
#8961=DIRECTION ( 'NONE',  ( 0.000000000000000000, -0.9612513907525602752, -0.2756732917354685064 ) ) ;
#8999=EDGE_CURVE ( 'NONE', #14199, #17744, #25339, .T. ) ;
#9005=CARTESIAN_POINT ( 'NONE',  ( 232.4999999999996305, 133.0668745871126930, -42.88984227207694744 ) ) ;
#9011=VERTEX_POINT ( 'NONE', #14571 ) ;
#9049=EDGE_LOOP ( 'NONE', ( #5045, #9127, #21873, #10647 ) ) ;
#9127=ORIENTED_EDGE ( 'NONE', *, *, #6544, .T. ) ;
#9128=CARTESIAN_POINT ( 'NONE',  ( 367.4999999999996021, 44.41075299063185611, -75.00000000000001421 ) ) ;
#9136=EDGE_CURVE ( 'NONE', #7154, #24450, #22600, .T. ) ;
#9188=PLANE ( 'NONE',  #1059 ) ;
#9239=LINE ( 'NONE', #7516, #4444 ) ;
#9245=VECTOR ( 'NONE', #74, 1000.000000000000000 ) ;
#9260=ORIENTED_EDGE ( 'NONE', *, *, #1977, .T. ) ;
#9277=VERTEX_POINT ( 'NONE', #5587 ) ;
#9340=CARTESIAN_POINT ( 'NONE',  ( 232.4999999999996305, 83.06687458711267880, -30.83984227207693607 ) ) ;
#9345=DIRECTION ( 'NONE',  ( 1.000000000000000000, -0.000000000000000000, -0.000000000000000000 ) ) ;
#9350=ORIENTED_EDGE ( 'NONE', *, *, #19705, .F. ) ;
#9351=AXIS2_PLACEMENT_3D ( 'NONE', #5047, #7504, #22587 ) ;
#9356=ORIENTED_EDGE ( 'NONE', *, *, #18501, .T. ) ;
#9432=VERTEX_POINT ( 'NONE', #4981 ) ;
#9436=EDGE_CURVE ( 'NONE', #20572, #21229, #3799, .T. ) ;
#9456=AXIS2_PLACEMENT_3D ( 'NONE', #8104, #5521, #1630 ) ;
#9522=ORIENTED_EDGE ( 'NONE', *, *, #27821, .T. ) ;
#9579=VECTOR ( 'NONE', #12937, 1000.000000000000000 ) ;
#9618=DIRECTION ( 'NONE',  ( 0.000000000000000000, 0.000000000000000000, -1.000000000000000000 ) ) ;
#9680=DIRECTION ( 'NONE',  ( 0.000000000000000000, 0.000000000000000000, -1.000000000000000000 ) ) ;
#9684=EDGE_LOOP ( 'NONE', ( #15667, #20286 ) ) ;
#9699=VECTOR ( 'NONE', #24842, 1000.000000000000000 ) ;
#9700=CARTESIAN_POINT ( 'NONE',  ( 502.4999999999996021, 494.4107529906318632, 75.35061095560301681 ) ) ;
#9716=EDGE_CURVE ( 'NONE', #8492, #26679, #21628, .T. ) ;
#9740=VERTEX_POINT ( 'NONE', #21201 ) ;
#9813=CIRCLE ( 'NONE', #14889, 6.025000000000002132 ) ;
#9830=VERTEX_POINT ( 'NONE', #13169 ) ;
#9862=CARTESIAN_POINT ( 'NONE',  ( 217.4999999999996305, 44.41075299063186321, -100.0000000000000142 ) ) ;
#9891=ADVANCED_FACE ( 'NONE', ( #24926 ), #16175, .T. ) ;
#9898=AXIS2_PLACEMENT_3D ( 'NONE', #13424, #11273, #2484 ) ;
#9950=VERTEX_POINT ( 'NONE', #2944 ) ;
#10053=ORIENTED_EDGE ( 'NONE', *, *, #19705, .T. ) ;
#10063=VECTOR ( 'NONE', #7250, 1000.000000000000000 ) ;
#10071=DIRECTION ( 'NONE',  ( 0.7071067811865474617, 0.000000000000000000, -0.7071067811865474617 ) ) ;
#10079=ORIENTED_EDGE ( 'NONE', *, *, #1360, .F. ) ;
#10086=EDGE_LOOP ( 'NONE', ( #7885, #14505, #2642, #13298 ) ) ;
#10099=ADVANCED_FACE ( 'NONE', ( #25755 ), #3923, .T. ) ;
#10127=CARTESIAN_POINT ( 'NONE',  ( 232.4999999999996305, 186.4134324495536248, 35.02193266779035952 ) ) ;
#10162=ORIENTED_EDGE ( 'NONE', *, *, #26141, .T. ) ;
#10197=PLANE ( 'NONE',  #27845 ) ;
#10211=DIRECTION ( 'NONE',  ( -0.000000000000000000, -9.208809080520486542E-17, 1.000000000000000000 ) ) ;
#10231=CARTESIAN_POINT ( 'NONE',  ( 432.4999999999996589, -5.589247009368160768, 100.0000000000000426 ) ) ;
#10241=VECTOR ( 'NONE', #5913, 1000.000000000000114 ) ;
#10248=DIRECTION ( 'NONE',  ( 1.000000000000000000, -0.000000000000000000, -0.000000000000000000 ) ) ;
#10258=DIRECTION ( 'NONE',  ( -1.000000000000000000, 0.000000000000000000, 0.000000000000000000 ) ) ;
#10312=EDGE_CURVE ( 'NONE', #16161, #19401, #3318, .T. ) ;
#10315=PLANE ( 'NONE',  #8782 ) ;
#10336=DIRECTION ( 'NONE',  ( 0.000000000000000000, -1.000000000000000000, -1.214306433183764966E-16 ) ) ;
#10341=CARTESIAN_POINT ( 'NONE',  ( 232.4999999999996305, 194.4107529906318064, -62.90796922943941638 ) ) ;
#10350=CARTESIAN_POINT ( 'NONE',  ( 372.9108539694884144, 19.41075299063184900, 87.99671038392668265 ) ) ;
#10355=VERTEX_POINT ( 'NONE', #1171 ) ;
#10357=ORIENTED_EDGE ( 'NONE', *, *, #8145, .F. ) ;
#10359=VECTOR ( 'NONE', #797, 1000.000000000000000 ) ;
#10367=EDGE_LOOP ( 'NONE', ( #1273, #1840, #27064, #8850 ) ) ;
#10369=DIRECTION ( 'NONE',  ( 1.000000000000000000, -0.000000000000000000, -0.000000000000000000 ) ) ;
#10384=DIRECTION ( 'NONE',  ( -1.000000000000000000, 0.000000000000000000, -0.000000000000000000 ) ) ;
#10415=CARTESIAN_POINT ( 'NONE',  ( 217.4999999999996305, 44.41075299063186321, -100.0000000000000142 ) ) ;
#10416=DIRECTION ( 'NONE',  ( 0.000000000000000000, 0.000000000000000000, 1.000000000000000000 ) ) ;
#10466=ORIENTED_EDGE ( 'NONE', *, *, #1064, .F. ) ;
#10467=ORIENTED_EDGE ( 'NONE', *, *, #9716, .F. ) ;
#10470=EDGE_LOOP ( 'NONE', ( #24824, #7295, #16, #17356 ) ) ;
#10481=CARTESIAN_POINT ( 'NONE',  ( 232.4749999999995964, 133.0668745871126930, -42.86484227207692044 ) ) ;
#10487=ADVANCED_FACE ( 'NONE', ( #19971 ), #21704, .T. ) ;
#10530=ORIENTED_EDGE ( 'NONE', *, *, #4874, .F. ) ;
#10536=VECTOR ( 'NONE', #6290, 1000.000000000000000 ) ;
#10551=EDGE_CURVE ( 'NONE', #26471, #12356, #4675, .T. ) ;
#10626=LINE ( 'NONE', #6024, #6191 ) ;
#10637=AXIS2_PLACEMENT_3D ( 'NONE', #25065, #2320, #14860 ) ;
#10643=ORIENTED_EDGE ( 'NONE', *, *, #21419, .F. ) ;
#10647=ORIENTED_EDGE ( 'NONE', *, *, #21691, .F. ) ;
#10649=EDGE_CURVE ( 'NONE', #16763, #20178, #24715, .T. ) ;
#10659=DIRECTION ( 'NONE',  ( 1.000000000000000000, -0.000000000000000000, -0.000000000000000000 ) ) ;
#10663=DIRECTION ( 'NONE',  ( 0.000000000000000000, 0.000000000000000000, -1.000000000000000000 ) ) ;
#10676=LINE ( 'NONE', #19433, #14241 ) ;
#10679=DIRECTION ( 'NONE',  ( 0.000000000000000000, 0.000000000000000000, -1.000000000000000000 ) ) ;
#10689=LINE ( 'NONE', #6652, #7190 ) ;
#10700=AXIS2_PLACEMENT_3D ( 'NONE', #24809, #20207, #11612 ) ;
#10706=DIRECTION ( 'NONE',  ( 0.000000000000000000, -1.000000000000000000, -1.214306433183764966E-16 ) ) ;
#10745=CONICAL_SURFACE ( 'NONE', #5261, 6.025000000000002132, 0.7853981633971707232 ) ;
#10747=DIRECTION ( 'NONE',  ( 1.000000000000000000, 0.000000000000000000, 0.000000000000000000 ) ) ;
#10793=EDGE_LOOP ( 'NONE', ( #28357, #2084, #5791, #21157 ) ) ;
#10837=DIRECTION ( 'NONE',  ( 1.000000000000000000, -0.000000000000000000, -0.000000000000000000 ) ) ;
#10889=EDGE_CURVE ( 'NONE', #15333, #9950, #598, .T. ) ;
#10923=ADVANCED_FACE ( 'NONE', ( #27502 ), #11625, .F. ) ;
#10944=VECTOR ( 'NONE', #20838, 1000.000000000000000 ) ;
#10952=CYLINDRICAL_SURFACE ( 'NONE', #2947, 100.0000000000000284 ) ;
#10993=FACE_OUTER_BOUND ( 'NONE', #1182, .T. ) ;
#11056=FACE_OUTER_BOUND ( 'NONE', #4449, .T. ) ;
#11066=AXIS2_PLACEMENT_3D ( 'NONE', #22252, #4328, #2563 ) ;
#11085=DIRECTION ( 'NONE',  ( -1.000000000000000000, 0.000000000000000000, -9.251858538542972814E-17 ) ) ;
#11093=CARTESIAN_POINT ( 'NONE',  ( 217.4999999999996305, 133.0668745871126930, -30.86484227207697018 ) ) ;
#11195=DIRECTION ( 'NONE',  ( 1.000000000000000000, -0.000000000000000000, -0.000000000000000000 ) ) ;
#11216=CARTESIAN_POINT ( 'NONE',  ( 222.4999999999996021, 186.4134324495536248, -35.02193266779035952 ) ) ;
#11225=CARTESIAN_POINT ( 'NONE',  ( 367.4999999999996021, 44.41075299063184190, 75.00000000000004263 ) ) ;
#11235=ADVANCED_FACE ( 'NONE', ( #27131, #20096, #11647, #22111, #13799 ), #9188, .T. ) ;
#11251=VERTEX_POINT ( 'NONE', #18935 ) ;
#11266=AXIS2_PLACEMENT_3D ( 'NONE', #25357, #4633, #198 ) ;
#11273=DIRECTION ( 'NONE',  ( 0.000000000000000000, -1.000000000000000000, -1.214306433183764966E-16 ) ) ;
#11285=DIRECTION ( 'NONE',  ( 0.000000000000000000, 0.000000000000000000, -1.000000000000000000 ) ) ;
#11301=ORIENTED_EDGE ( 'NONE', *, *, #12011, .F. ) ;
#11302=ORIENTED_EDGE ( 'NONE', *, *, #14715, .F. ) ;
#11340=EDGE_CURVE ( 'NONE', #4176, #16411, #14216, .T. ) ;
#11349=FACE_OUTER_BOUND ( 'NONE', #10367, .T. ) ;
#11354=LINE ( 'NONE', #22115, #13391 ) ;
#11358=VECTOR ( 'NONE', #16255, 999.9999999999998863 ) ;
#11362=ORIENTED_EDGE ( 'NONE', *, *, #4736, .T. ) ;
#11399=ORIENTED_EDGE ( 'NONE', *, *, #12095, .F. ) ;
#11404=CARTESIAN_POINT ( 'NONE',  ( 367.9108539694884144, 19.41075299063184900, 80.49671038392669686 ) ) ;
#11422=CARTESIAN_POINT ( 'NONE',  ( 367.4999999999996021, 44.41075299063184900, 1.850330238640837654E-14 ) ) ;
#11446=ORIENTED_EDGE ( 'NONE', *, *, #23057, .T. ) ;
#11522=DIRECTION ( 'NONE',  ( 1.000000000000000000, -0.000000000000000000, -0.000000000000000000 ) ) ;
#11529=AXIS2_PLACEMENT_3D ( 'NONE', #5316, #11522, #20260 ) ;
#11546=ORIENTED_EDGE ( 'NONE', *, *, #1096, .F. ) ;
#11548=EDGE_CURVE ( 'NONE', #26033, #15470, #15628, .T. ) ;
#11564=DIRECTION ( 'NONE',  ( 1.000000000000000000, -0.000000000000000000, -0.000000000000000000 ) ) ;
#11567=ORIENTED_EDGE ( 'NONE', *, *, #5559, .F. ) ;
#11577=CARTESIAN_POINT ( 'NONE',  ( 367.9108539694884144, 19.41075299063184900, 95.49671038392668265 ) ) ;
#11612=DIRECTION ( 'NONE',  ( 0.000000000000000000, 0.000000000000000000, 1.000000000000000000 ) ) ;
#11625=CONICAL_SURFACE ( 'NONE', #5627, 6.025000000000002132, 0.7853981633974482790 ) ;
#11647=FACE_BOUND ( 'NONE', #5902, .T. ) ;
#11648=EDGE_CURVE ( 'NONE', #11251, #8811, #20786, .T. ) ;
#11668=CYLINDRICAL_SURFACE ( 'NONE', #11529, 5.999999999999991118 ) ;
#11670=DIRECTION ( 'NONE',  ( 0.000000000000000000, 0.000000000000000000, -1.000000000000000000 ) ) ;
#11688=ORIENTED_EDGE ( 'NONE', *, *, #18445, .F. ) ;
#11703=CARTESIAN_POINT ( 'NONE',  ( 282.4999999999996589, 19.41075299063184900, 95.49671038392668265 ) ) ;
#11754=DIRECTION ( 'NONE',  ( 0.000000000000000000, 1.272130549049657961E-16, -1.000000000000000000 ) ) ;
#11774=EDGE_CURVE ( 'NONE', #12605, #2227, #819, .T. ) ;
#11780=CARTESIAN_POINT ( 'NONE',  ( 232.4999999999996305, 133.0668745871126930, -36.86484227207694886 ) ) ;
#11824=PRODUCT_CONTEXT ( 'NONE', #5981, 'mechanical' ) ;
#11843=DIRECTION ( 'NONE',  ( 1.000000000000000000, 0.000000000000000000, 0.000000000000000000 ) ) ;
#11853=EDGE_LOOP ( 'NONE', ( #5767, #22873, #26835, #23118 ) ) ;
#11883=CARTESIAN_POINT ( 'NONE',  ( 232.4999999999996305, 186.4134324495536248, -35.02193266779035952 ) ) ;
#11904=EDGE_LOOP ( 'NONE', ( #14370, #3929, #21484, #13605 ) ) ;
#11922=CARTESIAN_POINT ( 'NONE',  ( 232.4999999999996305, 133.0668745871126930, -36.86484227207694886 ) ) ;
#11932=VECTOR ( 'NONE', #14892, 1000.000000000000000 ) ;
#11948=CARTESIAN_POINT ( 'NONE',  ( 367.4999999999996021, 44.41075299063184900, 1.850330238640837654E-14 ) ) ;
#11952=DIRECTION ( 'NONE',  ( 0.000000000000000000, 1.024644424698391667E-16, -1.000000000000000000 ) ) ;
#11954=DIRECTION ( 'NONE',  ( 0.000000000000000000, 0.000000000000000000, 1.000000000000000000 ) ) ;
#12009=CIRCLE ( 'NONE', #53, 5.999999999999977796 ) ;
#12011=EDGE_CURVE ( 'NONE', #26013, #15680, #21899, .T. ) ;
#12051=DIRECTION ( 'NONE',  ( -1.000000000000000000, 0.000000000000000000, -0.000000000000000000 ) ) ;
#12068=CARTESIAN_POINT ( 'NONE',  ( 367.9108539694884144, 44.41075299063183479, 100.0000000000000284 ) ) ;
#12077=VERTEX_POINT ( 'NONE', #24199 ) ;
#12095=EDGE_CURVE ( 'NONE', #10355, #12452, #8446, .T. ) ;
#12115=DIRECTION ( 'NONE',  ( 0.000000000000000000, -1.000000000000000000, 0.000000000000000000 ) ) ;
#12144=CARTESIAN_POINT ( 'NONE',  ( 372.9108539694884144, -5.589247009368157215, 74.80456309157131045 ) ) ;
#12167=DIRECTION ( 'NONE',  ( 0.000000000000000000, 9.251858538542967883E-17, -1.000000000000000000 ) ) ;
#12205=DIRECTION ( 'NONE',  ( -0.000000000000000000, -0.000000000000000000, 1.000000000000000000 ) ) ;
#12215=AXIS2_PLACEMENT_3D ( 'NONE', #21757, #8961, #4636 ) ;
#12231=EDGE_CURVE ( 'NONE', #12519, #506, #27200, .T. ) ;
#12260=VERTEX_POINT ( 'NONE', #18584 ) ;
#12341=CARTESIAN_POINT ( 'NONE',  ( 367.9108539694884144, 44.41075299063184190, 74.99887465166234790 ) ) ;
#12355=ORIENTED_EDGE ( 'NONE', *, *, #4980, .T. ) ;
#12356=VERTEX_POINT ( 'NONE', #14990 ) ;
#12366=ADVANCED_FACE ( 'NONE', ( #3909 ), #25468, .F. ) ;
#12389=EDGE_CURVE ( 'NONE', #20612, #26679, #8090, .T. ) ;
#12399=CARTESIAN_POINT ( 'NONE',  ( 217.4999999999996305, 133.0668745871126930, -36.86484227207694886 ) ) ;
#12404=DIRECTION ( 'NONE',  ( 1.000000000000000000, -0.000000000000000000, -0.000000000000000000 ) ) ;
#12452=VERTEX_POINT ( 'NONE', #13123 ) ;
#12498=EDGE_LOOP ( 'NONE', ( #2465, #24607, #27967, #14361 ) ) ;
#12506=VECTOR ( 'NONE', #25449, 1000.000000000000000 ) ;
#12511=FACE_BOUND ( 'NONE', #12636, .T. ) ;
#12512=LINE ( 'NONE', #12790, #16095 ) ;
#12519=VERTEX_POINT ( 'NONE', #13543 ) ;
#12526=VERTEX_POINT ( 'NONE', #11093 ) ;
#12538=ADVANCED_FACE ( 'NONE', ( #13398 ), #10952, .T. ) ;
#12573=DIRECTION ( 'NONE',  ( -0.000000000000000000, -0.3247168404252948060, -0.9458112779747414045 ) ) ;
#12605=VERTEX_POINT ( 'NONE', #19848 ) ;
#12636=EDGE_LOOP ( 'NONE', ( #23227, #11302 ) ) ;
#12671=ORIENTED_EDGE ( 'NONE', *, *, #6037, .T. ) ;
#12707=DIRECTION ( 'NONE',  ( 0.000000000000000000, 9.251858538542967883E-17, -1.000000000000000000 ) ) ;
#12720=EDGE_CURVE ( 'NONE', #12356, #26471, #20841, .T. ) ;
#12734=ORIENTED_EDGE ( 'NONE', *, *, #15590, .F. ) ;
#12744=ADVANCED_FACE ( 'NONE', ( #21942 ), #10745, .F. ) ;
#12790=CARTESIAN_POINT ( 'NONE',  ( 367.4999999999996021, 44.41075299063184190, 75.00000000000004263 ) ) ;
#12801=ORIENTED_EDGE ( 'NONE', *, *, #12720, .F. ) ;
#12816=EDGE_LOOP ( 'NONE', ( #16928, #10079, #14793, #19826 ) ) ;
#12819=CONICAL_SURFACE ( 'NONE', #13268, 6.025000000000002132, 0.7853981633974482790 ) ;
#12826=CARTESIAN_POINT ( 'NONE',  ( 330.9869376377542949, 44.41075299063183479, 100.0000000000000284 ) ) ;
#12859=AXIS2_PLACEMENT_3D ( 'NONE', #16463, #27496, #1644 ) ;
#12861=DIRECTION ( 'NONE',  ( 0.000000000000000000, 0.000000000000000000, -1.000000000000000000 ) ) ;
#12862=PLANE ( 'NONE',  #12215 ) ;
#12905=CARTESIAN_POINT ( 'NONE',  ( 232.4749999999995964, 133.0668745871126930, -30.86484227207697018 ) ) ;
#12924=VERTEX_POINT ( 'NONE', #17917 ) ;
#12936=CIRCLE ( 'NONE', #14783, 5.999999999999991118 ) ;
#12937=DIRECTION ( 'NONE',  ( 1.000000000000000000, -0.000000000000000000, -0.000000000000000000 ) ) ;
#12949=SHAPE_DEFINITION_REPRESENTATION ( #27675, #22013 ) ;
#12970=AXIS2_PLACEMENT_3D ( 'NONE', #3215, #5938, #12707 ) ;
#12971=EDGE_CURVE ( 'NONE', #9432, #21245, #4833, .T. ) ;
#13003=ORIENTED_EDGE ( 'NONE', *, *, #23739, .F. ) ;
#13025=DIRECTION ( 'NONE',  ( 0.000000000000000000, 0.000000000000000000, -1.000000000000000000 ) ) ;
#13054=DIRECTION ( 'NONE',  ( 0.000000000000000000, 0.000000000000000000, 1.000000000000000000 ) ) ;
#13067=LINE ( 'NONE', #4555, #15529 ) ;
#13102=CARTESIAN_POINT ( 'NONE',  ( 217.4999999999996305, 83.06687458711267880, -36.86484227207694175 ) ) ;
#13120=VECTOR ( 'NONE', #7237, 1000.000000000000000 ) ;
#13123=CARTESIAN_POINT ( 'NONE',  ( 432.4999999999996589, 19.41075299063184900, 80.49671038392669686 ) ) ;
#13169=CARTESIAN_POINT ( 'NONE',  ( 432.4999999999996589, -5.589247009368160768, 100.0000000000000426 ) ) ;
#13206=ORIENTED_EDGE ( 'NONE', *, *, #26141, .F. ) ;
#13213=ADVANCED_FACE ( 'NONE', ( #3951 ), #21478, .F. ) ;
#13224=LINE ( 'NONE', #19675, #9579 ) ;
#13268=AXIS2_PLACEMENT_3D ( 'NONE', #214, #17447, #19743 ) ;
#13279=VECTOR ( 'NONE', #2130, 1000.000000000000000 ) ;
#13298=ORIENTED_EDGE ( 'NONE', *, *, #16939, .F. ) ;
#13301=ORIENTED_EDGE ( 'NONE', *, *, #10312, .T. ) ;
#13371=VECTOR ( 'NONE', #17263, 1000.000000000000000 ) ;
#13391=VECTOR ( 'NONE', #6738, 1000.000000000000000 ) ;
#13398=FACE_OUTER_BOUND ( 'NONE', #26529, .T. ) ;
#13415=ORIENTED_EDGE ( 'NONE', *, *, #17947, .T. ) ;
#13420=FACE_OUTER_BOUND ( 'NONE', #17749, .T. ) ;
#13424=CARTESIAN_POINT ( 'NONE',  ( 367.4999999999996021, -5.589247009368149222, 1.243177022048955014E-14 ) ) ;
#13442=VERTEX_POINT ( 'NONE', #12144 ) ;
#13446=ORIENTED_EDGE ( 'NONE', *, *, #24177, .F. ) ;
#13450=EDGE_CURVE ( 'NONE', #21245, #5808, #7543, .T. ) ;
#13459=AXIS2_PLACEMENT_3D ( 'NONE', #9700, #18461, #5241 ) ;
#13468=DIRECTION ( 'NONE',  ( 0.000000000000000000, -1.000000000000000000, -1.214306433183764966E-16 ) ) ;
#13498=DIRECTION ( 'NONE',  ( 0.000000000000000000, 0.000000000000000000, -1.000000000000000000 ) ) ;
#13518=AXIS2_PLACEMENT_3D ( 'NONE', #21580, #15129, #27751 ) ;
#13541=CARTESIAN_POINT ( 'NONE',  ( 232.4999999999996305, 83.06687458711267880, -36.86484227207694175 ) ) ;
#13543=CARTESIAN_POINT ( 'NONE',  ( 222.4999999999996021, 194.4107529906318064, 58.31593845887894645 ) ) ;
#13589=LINE ( 'NONE', #20468, #8785 ) ;
#13602=EDGE_CURVE ( 'NONE', #12452, #10355, #1154, .T. ) ;
#13605=ORIENTED_EDGE ( 'NONE', *, *, #3401, .T. ) ;
#13613=DIRECTION ( 'NONE',  ( 0.000000000000000000, 0.000000000000000000, 1.000000000000000000 ) ) ;
#13621=CARTESIAN_POINT ( 'NONE',  ( 367.4999999999996021, 44.41075299063184900, 1.850330238640837654E-14 ) ) ;
#13622=EDGE_CURVE ( 'NONE', #23606, #19624, #469, .T. ) ;
#13772=AXIS2_PLACEMENT_3D ( 'NONE', #10350, #5614, #7775 ) ;
#13780=ORIENTED_EDGE ( 'NONE', *, *, #18540, .T. ) ;
#13792=PLANE ( 'NONE',  #14165 ) ;
#13799=FACE_OUTER_BOUND ( 'NONE', #27082, .T. ) ;
#13813=VECTOR ( 'NONE', #913, 1000.000000000000114 ) ;
#13835=FACE_OUTER_BOUND ( 'NONE', #6047, .T. ) ;
#13836=VECTOR ( 'NONE', #11952, 1000.000000000000000 ) ;
#13871=ORIENTED_EDGE ( 'NONE', *, *, #18128, .F. ) ;
#13881=ORIENTED_EDGE ( 'NONE', *, *, #25090, .F. ) ;
#13890=CARTESIAN_POINT ( 'NONE',  ( 232.4749999999995964, 133.0668745871126930, 36.86484227207694886 ) ) ;
#13913=CARTESIAN_POINT ( 'NONE',  ( 217.4999999999996305, 44.41075299063183479, 100.0000000000000142 ) ) ;
#13925=ORIENTED_EDGE ( 'NONE', *, *, #4980, .F. ) ;
#13935=DIRECTION ( 'NONE',  ( 0.3897722486529259234, -0.9209112846414913012, -1.118268497331688440E-16 ) ) ;
#13936=AXIS2_PLACEMENT_3D ( 'NONE', #1739, #10659, #14977 ) ;
#13939=CARTESIAN_POINT ( 'NONE',  ( 367.4999999999996021, 44.41075299063183479, 100.0000000000000284 ) ) ;
#13961=CARTESIAN_POINT ( 'NONE',  ( 372.9108539694884144, -5.589247009368160768, 100.0000000000000426 ) ) ;
#13988=ADVANCED_FACE ( 'NONE', ( #2431 ), #19685, .F. ) ;
#13992=EDGE_LOOP ( 'NONE', ( #16519, #1417, #3681, #25162 ) ) ;
#14009=PLANE ( 'NONE',  #14144 ) ;
#14041=CIRCLE ( 'NONE', #2543, 5.999999999999991118 ) ;
#14081=ADVANCED_FACE ( 'NONE', ( #13420 ), #12862, .F. ) ;
#14090=VECTOR ( 'NONE', #12573, 1000.000000000000000 ) ;
#14094=ORIENTED_EDGE ( 'NONE', *, *, #12095, .T. ) ;
#14098=DIRECTION ( 'NONE',  ( 0.000000000000000000, 0.000000000000000000, -1.000000000000000000 ) ) ;
#14121=ORIENTED_EDGE ( 'NONE', *, *, #16816, .T. ) ;
#14125=DIRECTION ( 'NONE',  ( 1.000000000000000000, -0.000000000000000000, -0.000000000000000000 ) ) ;
#14136=CARTESIAN_POINT ( 'NONE',  ( 372.9108539694884144, 19.41075299063184900, 95.49671038392668265 ) ) ;
#14144=AXIS2_PLACEMENT_3D ( 'NONE', #11422, #496, #4788 ) ;
#14150=ORIENTED_EDGE ( 'NONE', *, *, #7076, .T. ) ;
#14165=AXIS2_PLACEMENT_3D ( 'NONE', #22686, #19948, #22539 ) ;
#14168=EDGE_CURVE ( 'NONE', #16763, #23612, #14041, .T. ) ;
#14174=CARTESIAN_POINT ( 'NONE',  ( 232.4999999999996305, 133.0668745871126930, 36.86484227207694886 ) ) ;
#14199=VERTEX_POINT ( 'NONE', #26194 ) ;
#14216=LINE ( 'NONE', #24982, #1529 ) ;
#14229=ORIENTED_EDGE ( 'NONE', *, *, #3549, .F. ) ;
#14236=DIRECTION ( 'NONE',  ( 0.000000000000000000, 0.000000000000000000, 1.000000000000000000 ) ) ;
#14241=VECTOR ( 'NONE', #23461, 1000.000000000000000 ) ;
#14245=FACE_BOUND ( 'NONE', #24962, .T. ) ;
#14279=VECTOR ( 'NONE', #10071, 1000.000000000000114 ) ;
#14284=CARTESIAN_POINT ( 'NONE',  ( 232.4999999999996305, 83.06687458711267880, 30.83984227207693607 ) ) ;
#14354=AXIS2_PLACEMENT_3D ( 'NONE', #12399, #28014, #21135 ) ;
#14356=DIRECTION ( 'NONE',  ( 0.000000000000000000, -1.000000000000000000, -1.214306433183764966E-16 ) ) ;
#14358=EDGE_CURVE ( 'NONE', #20612, #9432, #283, .T. ) ;
#14361=ORIENTED_EDGE ( 'NONE', *, *, #3832, .F. ) ;
#14370=ORIENTED_EDGE ( 'NONE', *, *, #26305, .F. ) ;
#14443=LINE ( 'NONE', #10127, #14090 ) ;
#14457=FACE_OUTER_BOUND ( 'NONE', #9049, .T. ) ;
#14483=LINE ( 'NONE', #5419, #7484 ) ;
#14505=ORIENTED_EDGE ( 'NONE', *, *, #8145, .T. ) ;
#14523=DIRECTION ( 'NONE',  ( 0.000000000000000000, 0.000000000000000000, -1.000000000000000000 ) ) ;
#14571=CARTESIAN_POINT ( 'NONE',  ( 367.9108539694884144, 44.41075299063183479, 100.0000000000000284 ) ) ;
#14584=LINE ( 'NONE', #6091, #28106 ) ;
#14592=EDGE_CURVE ( 'NONE', #8019, #18668, #27955, .T. ) ;
#14621=VECTOR ( 'NONE', #28245, 1000.000000000000000 ) ;
#14634=LINE ( 'NONE', #12068, #15120 ) ;
#14660=PLANE ( 'NONE',  #8187 ) ;
#14681=CIRCLE ( 'NONE', #5957, 7.499999999999992895 ) ;
#14686=DIRECTION ( 'NONE',  ( 1.000000000000000000, -0.000000000000000000, -0.000000000000000000 ) ) ;
#14690=CARTESIAN_POINT ( 'NONE',  ( 232.4749999999995964, 83.06687458711267880, -42.86484227207692754 ) ) ;
#14697=EDGE_CURVE ( 'NONE', #9432, #16411, #19772, .T. ) ;
#14714=EDGE_CURVE ( 'NONE', #7154, #25274, #8721, .T. ) ;
#14715=EDGE_CURVE ( 'NONE', #17607, #23614, #24155, .T. ) ;
#14783=AXIS2_PLACEMENT_3D ( 'NONE', #23598, #10248, #21434 ) ;
#14793=ORIENTED_EDGE ( 'NONE', *, *, #6294, .F. ) ;
#14804=DIRECTION ( 'NONE',  ( -0.000000000000000000, 0.2756732917354685064, -0.9612513907525602752 ) ) ;
#14812=DIRECTION ( 'NONE',  ( 0.000000000000000000, -1.000000000000000000, -1.214306433183764966E-16 ) ) ;
#14846=ORIENTED_EDGE ( 'NONE', *, *, #23003, .F. ) ;
#14851=DIRECTION ( 'NONE',  ( 0.000000000000000000, 0.000000000000000000, -1.000000000000000000 ) ) ;
#14860=DIRECTION ( 'NONE',  ( 1.000000000000000000, 0.000000000000000000, 0.000000000000000000 ) ) ;
#14886=DIRECTION ( 'NONE',  ( 0.000000000000000000, 1.214306433183764720E-16, -1.000000000000000000 ) ) ;
#14888=ORIENTED_EDGE ( 'NONE', *, *, #7440, .F. ) ;
#14889=AXIS2_PLACEMENT_3D ( 'NONE', #4567, #19379, #28130 ) ;
#14892=DIRECTION ( 'NONE',  ( 0.000000000000000000, -1.000000000000000000, -1.214306433183764966E-16 ) ) ;
#14977=DIRECTION ( 'NONE',  ( 0.000000000000000000, 0.000000000000000000, -1.000000000000000000 ) ) ;
#14988=CARTESIAN_POINT ( 'NONE',  ( 232.4999999999996305, 83.06687458711267880, -30.86484227207694886 ) ) ;
#14990=CARTESIAN_POINT ( 'NONE',  ( 217.4999999999996305, 83.06687458711267880, -30.86484227207694886 ) ) ;
#15013=FACE_OUTER_BOUND ( 'NONE', #2783, .T. ) ;
#15014=CARTESIAN_POINT ( 'NONE',  ( 232.4749999999995964, 83.06687458711267880, -36.86484227207694175 ) ) ;
#15052=DIRECTION ( 'NONE',  ( 0.000000000000000000, -1.000000000000000000, -1.214306433183764966E-16 ) ) ;
#15055=PLANE ( 'NONE',  #21938 ) ;
#15059=EDGE_CURVE ( 'NONE', #8019, #26636, #5339, .T. ) ;
#15106=DIRECTION ( 'NONE',  ( 0.000000000000000000, -1.000000000000000000, -1.214306433183764966E-16 ) ) ;
#15120=VECTOR ( 'NONE', #14356, 1000.000000000000000 ) ;
#15129=DIRECTION ( 'NONE',  ( 0.000000000000000000, -1.000000000000000000, -1.214306433183764966E-16 ) ) ;
#15203=EDGE_CURVE ( 'NONE', #2227, #26033, #19192, .T. ) ;
#15205=FACE_OUTER_BOUND ( 'NONE', #2825, .T. ) ;
#15217=ORIENTED_EDGE ( 'NONE', *, *, #25952, .T. ) ;
#15266=CARTESIAN_POINT ( 'NONE',  ( 367.4999999999996021, -5.589247009368160768, 100.0000000000000284 ) ) ;
#15278=VECTOR ( 'NONE', #24686, 1000.000000000000000 ) ;
#15295=ADVANCED_FACE ( 'NONE', ( #3201 ), #14009, .F. ) ;
#15311=CARTESIAN_POINT ( 'NONE',  ( 367.4999999999996021, -5.589247009368149222, 1.243177022048955014E-14 ) ) ;
#15327=ORIENTED_EDGE ( 'NONE', *, *, #23166, .F. ) ;
#15333=VERTEX_POINT ( 'NONE', #20309 ) ;
#15338=DIRECTION ( 'NONE',  ( 1.000000000000000000, -0.000000000000000000, -0.000000000000000000 ) ) ;
#15389=DIRECTION ( 'NONE',  ( -0.000000000000000000, 1.000000000000000000, 1.214306433183764966E-16 ) ) ;
#15431=ORIENTED_EDGE ( 'NONE', *, *, #26771, .F. ) ;
#15453=CARTESIAN_POINT ( 'NONE',  ( 232.4749999999995964, 83.06687458711267880, 30.86484227207694886 ) ) ;
#15470=VERTEX_POINT ( 'NONE', #7669 ) ;
#15473=ORIENTED_EDGE ( 'NONE', *, *, #743, .F. ) ;
#15484=CARTESIAN_POINT ( 'NONE',  ( 217.4999999999996305, 194.4107529906318064, 288.0938197134494203 ) ) ;
#15485=CARTESIAN_POINT ( 'NONE',  ( 232.4749999999995964, 83.06687458711267880, 42.86484227207692754 ) ) ;
#15490=CYLINDRICAL_SURFACE ( 'NONE', #21128, 75.00000000000002842 ) ;
#15511=DIRECTION ( 'NONE',  ( -0.000000000000000000, 0.000000000000000000, 1.000000000000000000 ) ) ;
#15526=ORIENTED_EDGE ( 'NONE', *, *, #7440, .T. ) ;
#15529=VECTOR ( 'NONE', #262, 1000.000000000000000 ) ;
#15545=CARTESIAN_POINT ( 'NONE',  ( 282.4999999999996589, 19.41075299063184900, 87.99671038392668265 ) ) ;
#15568=EDGE_LOOP ( 'NONE', ( #7893, #7952, #5306, #14888 ) ) ;
#15590=EDGE_CURVE ( 'NONE', #16161, #24580, #20092, .T. ) ;
#15600=DIRECTION ( 'NONE',  ( 1.000000000000000000, -0.000000000000000000, -0.000000000000000000 ) ) ;
#15624=DIRECTION ( 'NONE',  ( 0.7071067811865474617, 0.000000000000000000, -0.7071067811865474617 ) ) ;
#15628=LINE ( 'NONE', #251, #7026 ) ;
#15631=EDGE_CURVE ( 'NONE', #12077, #9740, #26308, .T. ) ;
#15667=ORIENTED_EDGE ( 'NONE', *, *, #3401, .F. ) ;
#15680=VERTEX_POINT ( 'NONE', #7496 ) ;
#15756=CARTESIAN_POINT ( 'NONE',  ( 432.4999999999996589, 44.41075299063185611, 75.99342076785332267 ) ) ;
#15775=DIRECTION ( 'NONE',  ( 0.000000000000000000, -1.000000000000000000, -1.214306433183764966E-16 ) ) ;
#15788=ADVANCED_FACE ( 'NONE', ( #1579 ), #14660, .T. ) ;
#15790=EDGE_LOOP ( 'NONE', ( #26219, #23682, #7651, #5810, #10530, #6686, #21372, #27683, #16424, #28104, #22585, #7553, #5120, #629, #18141 ) ) ;
#15798=FACE_OUTER_BOUND ( 'NONE', #6894, .T. ) ;
#15804=CARTESIAN_POINT ( 'NONE',  ( 367.4999999999996021, 44.41075299063185611, -75.00000000000001421 ) ) ;
#15833=EDGE_CURVE ( 'NONE', #26033, #25738, #21258, .T. ) ;
#15840=LINE ( 'NONE', #15266, #28163 ) ;
#15876=LINE ( 'NONE', #776, #13813 ) ;
#15924=DIRECTION ( 'NONE',  ( -0.3897722486529259234, 0.9209112846414913012, 1.118268497331688440E-16 ) ) ;
#15927=EDGE_CURVE ( 'NONE', #8811, #24580, #13224, .T. ) ;
#15928=DIRECTION ( 'NONE',  ( 0.000000000000000000, 0.000000000000000000, 1.000000000000000000 ) ) ;
#15973=DIRECTION ( 'NONE',  ( 0.000000000000000000, 0.000000000000000000, -1.000000000000000000 ) ) ;
#15989=DIRECTION ( 'NONE',  ( -0.9209112846414913012, -0.3897722486529259789, 0.000000000000000000 ) ) ;
#16013=CARTESIAN_POINT ( 'NONE',  ( 232.4999999999996305, 83.06687458711267880, -42.86484227207692754 ) ) ;
#16072=AXIS2_PLACEMENT_3D ( 'NONE', #11780, #11195, #13498 ) ;
#16074=VECTOR ( 'NONE', #20637, 1000.000000000000000 ) ;
#16095=VECTOR ( 'NONE', #4430, 1000.000000000000000 ) ;
#16161=VERTEX_POINT ( 'NONE', #15453 ) ;
#16175=PLANE ( 'NONE',  #13459 ) ;
#16199=DIRECTION ( 'NONE',  ( 1.000000000000000000, -0.000000000000000000, -0.000000000000000000 ) ) ;
#16251=ADVANCED_FACE ( 'NONE', ( #10993 ), #12819, .F. ) ;
#16255=DIRECTION ( 'NONE',  ( -0.3897722486529259234, 0.9209112846414913012, 7.576567266530214112E-17 ) ) ;
#16261=VECTOR ( 'NONE', #13935, 999.9999999999998863 ) ;
#16326=VECTOR ( 'NONE', #20628, 1000.000000000000000 ) ;
#16371=LINE ( 'NONE', #20948, #6322 ) ;
#16379=ORIENTED_EDGE ( 'NONE', *, *, #7865, .T. ) ;
#16395=EDGE_CURVE ( 'NONE', #2018, #12452, #26926, .T. ) ;
#16411=VERTEX_POINT ( 'NONE', #3065 ) ;
#16414=CARTESIAN_POINT ( 'NONE',  ( 232.4999999999996305, 83.06687458711267880, 30.83984227207693607 ) ) ;
#16422=EDGE_LOOP ( 'NONE', ( #20899, #17493, #22943, #16754 ) ) ;
#16424=ORIENTED_EDGE ( 'NONE', *, *, #18501, .F. ) ;
#16434=CONICAL_SURFACE ( 'NONE', #27417, 6.025000000000002132, 0.7853981633974482790 ) ;
#16451=CYLINDRICAL_SURFACE ( 'NONE', #9456, 5.999999999999977796 ) ;
#16463=CARTESIAN_POINT ( 'NONE',  ( 232.4749999999995964, 133.0668745871126930, -36.86484227207694886 ) ) ;
#16499=CIRCLE ( 'NONE', #21998, 6.025000000000002132 ) ;
#16508=CARTESIAN_POINT ( 'NONE',  ( 232.4999999999996305, 133.0668745871126930, -36.86484227207694886 ) ) ;
#16519=ORIENTED_EDGE ( 'NONE', *, *, #11648, .T. ) ;
#16596=EDGE_LOOP ( 'NONE', ( #14121, #762 ) ) ;
#16673=FACE_OUTER_BOUND ( 'NONE', #16422, .T. ) ;
#16676=LINE ( 'NONE', #6030, #863 ) ;
#16694=ORIENTED_EDGE ( 'NONE', *, *, #21674, .T. ) ;
#16754=ORIENTED_EDGE ( 'NONE', *, *, #17891, .T. ) ;
#16763=VERTEX_POINT ( 'NONE', #17989 ) ;
#16778=CARTESIAN_POINT ( 'NONE',  ( 367.4999999999996021, -5.589247009368149222, 1.243177022048955014E-14 ) ) ;
#16790=ADVANCED_FACE ( 'NONE', ( #13835 ), #2748, .F. ) ;
#16816=EDGE_CURVE ( 'NONE', #2018, #23487, #26127, .T. ) ;
#16818=PLANE ( 'NONE',  #3262 ) ;
#16873=ORIENTED_EDGE ( 'NONE', *, *, #8413, .F. ) ;
#16928=ORIENTED_EDGE ( 'NONE', *, *, #23166, .T. ) ;
#16939=EDGE_CURVE ( 'NONE', #13442, #8669, #21974, .T. ) ;
#16962=EDGE_LOOP ( 'NONE', ( #18844, #368, #3942, #399 ) ) ;
#17009=ORIENTED_EDGE ( 'NONE', *, *, #3832, .T. ) ;
#17028=CARTESIAN_POINT ( 'NONE',  ( 282.4999999999996589, 19.41075299063184900, 95.49671038392668265 ) ) ;
#17070=ORIENTED_EDGE ( 'NONE', *, *, #18399, .F. ) ;
#17096=DIRECTION ( 'NONE',  ( 0.000000000000000000, 1.214306433183764966E-16, -1.000000000000000000 ) ) ;
#17152=AXIS2_PLACEMENT_3D ( 'NONE', #26782, #6949, #499 ) ;
#17201=FACE_BOUND ( 'NONE', #8084, .T. ) ;
#17212=CIRCLE ( 'NONE', #18121, 75.00000000000002842 ) ;
#17248=ORIENTED_EDGE ( 'NONE', *, *, #19529, .T. ) ;
#17263=DIRECTION ( 'NONE',  ( -0.000000000000000000, -0.000000000000000000, -1.000000000000000000 ) ) ;
#17351=ORIENTED_EDGE ( 'NONE', *, *, #15203, .T. ) ;
#17356=ORIENTED_EDGE ( 'NONE', *, *, #24112, .T. ) ;
#17365=PLANE ( 'NONE',  #7619 ) ;
#17384=EDGE_CURVE ( 'NONE', #24450, #7154, #19729, .T. ) ;
#17447=DIRECTION ( 'NONE',  ( 1.000000000000000000, -0.000000000000000000, -0.000000000000000000 ) ) ;
#17486=VERTEX_POINT ( 'NONE', #1542 ) ;
#17493=ORIENTED_EDGE ( 'NONE', *, *, #12971, .F. ) ;
#17498=VECTOR ( 'NONE', #15924, 999.9999999999998863 ) ;
#17506=DIRECTION ( 'NONE',  ( -1.000000000000000000, 0.000000000000000000, -9.251858538542974046E-17 ) ) ;
#17524=DIRECTION ( 'NONE',  ( 0.000000000000000000, -0.000000000000000000, -1.000000000000000000 ) ) ;
#17569=ORIENTED_EDGE ( 'NONE', *, *, #10889, .T. ) ;
#17591=LINE ( 'NONE', #28348, #11932 ) ;
#17593=LINE ( 'NONE', #1794, #9245 ) ;
#17607=VERTEX_POINT ( 'NONE', #4398 ) ;
#17630=DIRECTION ( 'NONE',  ( 0.000000000000000000, -1.000000000000000000, -1.214306433183764966E-16 ) ) ;
#17632=CARTESIAN_POINT ( 'NONE',  ( 232.4999999999996305, 83.06687458711267880, 36.86484227207694175 ) ) ;
#17647=DIRECTION ( 'NONE',  ( 1.000000000000000000, -0.000000000000000000, -0.000000000000000000 ) ) ;
#17652=DIRECTION ( 'NONE',  ( 0.000000000000000000, 0.000000000000000000, -1.000000000000000000 ) ) ;
#17665=ORIENTED_EDGE ( 'NONE', *, *, #11774, .T. ) ;
#17688=CARTESIAN_POINT ( 'NONE',  ( 232.4999999999996305, 133.0668745871126930, 30.83984227207694317 ) ) ;
#17724=CARTESIAN_POINT ( 'NONE',  ( 217.4999999999996305, 133.0668745871126930, -42.86484227207692044 ) ) ;
#17744=VERTEX_POINT ( 'NONE', #7277 ) ;
#17749=EDGE_LOOP ( 'NONE', ( #13415, #18899, #25581, #5897 ) ) ;
#17768=DIRECTION ( 'NONE',  ( 0.000000000000000000, -1.000000000000000000, -1.214306433183764966E-16 ) ) ;
#17884=( LENGTH_UNIT ( ) NAMED_UNIT ( * ) SI_UNIT ( .MILLI., .METRE. ) );
#17886=ORIENTED_EDGE ( 'NONE', *, *, #11548, .T. ) ;
#17891=EDGE_CURVE ( 'NONE', #16411, #5808, #23345, .T. ) ;
#17907=DIRECTION ( 'NONE',  ( -1.000000000000000000, 0.000000000000000000, -0.000000000000000000 ) ) ;
#17917=CARTESIAN_POINT ( 'NONE',  ( 232.4999999999996305, 186.4134324495536248, 35.02193266779035952 ) ) ;
#17920=VECTOR ( 'NONE', #2173, 1000.000000000000000 ) ;
#17944=CYLINDRICAL_SURFACE ( 'NONE', #11066, 5.999999999999991118 ) ;
#17947=EDGE_CURVE ( 'NONE', #9277, #24079, #25771, .T. ) ;
#17949=CYLINDRICAL_SURFACE ( 'NONE', #1790, 5.999999999999991118 ) ;
#17957=DIRECTION ( 'NONE',  ( 0.000000000000000000, -1.000000000000000000, 0.000000000000000000 ) ) ;
#17977=DIRECTION ( 'NONE',  ( 1.000000000000000000, -0.000000000000000000, -0.000000000000000000 ) ) ;
#17989=CARTESIAN_POINT ( 'NONE',  ( 232.4749999999995964, 83.06687458711267880, -30.86484227207694886 ) ) ;
#18010=CARTESIAN_POINT ( 'NONE',  ( 372.9108539694884144, 19.41075299063184900, 80.49671038392669686 ) ) ;
#18073=ORIENTED_EDGE ( 'NONE', *, *, #2936, .F. ) ;
#18121=AXIS2_PLACEMENT_3D ( 'NONE', #11948, #25141, #24729 ) ;
#18127=ORIENTED_EDGE ( 'NONE', *, *, #7624, .F. ) ;
#18128=EDGE_CURVE ( 'NONE', #24580, #7480, #15876, .T. ) ;
#18139=SHAPE_REPRESENTATION_RELATIONSHIP ( 'NONE' , 'NONE' ,  #22013, #5057 ) ;
#18141=ORIENTED_EDGE ( 'NONE', *, *, #27794, .F. ) ;
#18159=AXIS2_PLACEMENT_3D ( 'NONE', #27641, #21184, #10416 ) ;
#18186=VECTOR ( 'NONE', #1122, 1000.000000000000000 ) ;
#18191=CARTESIAN_POINT ( 'NONE',  ( 222.4999999999996021, 186.4134324495536248, 35.02193266779035952 ) ) ;
#18224=EDGE_LOOP ( 'NONE', ( #16379, #13780, #3571, #21878 ) ) ;
#18242=LINE ( 'NONE', #24706, #8848 ) ;
#18259=VECTOR ( 'NONE', #12205, 1000.000000000000000 ) ;
#18327=ORIENTED_EDGE ( 'NONE', *, *, #3865, .F. ) ;
#18367=DIRECTION ( 'NONE',  ( 1.000000000000000000, -0.000000000000000000, -0.000000000000000000 ) ) ;
#18376=ADVANCED_FACE ( 'NONE', ( #11349 ), #17944, .F. ) ;
#18399=EDGE_CURVE ( 'NONE', #12077, #4176, #8510, .T. ) ;
#18404=CARTESIAN_POINT ( 'NONE',  ( 267.4999999999996021, 194.4107529906318064, -100.0000000000000000 ) ) ;
#18425=AXIS2_PLACEMENT_3D ( 'NONE', #26955, #16199, #25085 ) ;
#18445=EDGE_CURVE ( 'NONE', #23757, #26144, #7405, .T. ) ;
#18451=PRODUCT_DEFINITION ( 'UNKNOWN', '', #1929, #274 ) ;
#18461=DIRECTION ( 'NONE',  ( 0.000000000000000000, 1.214306433183764966E-16, -1.000000000000000000 ) ) ;
#18501=EDGE_CURVE ( 'NONE', #14199, #12605, #3414, .T. ) ;
#18520=FACE_OUTER_BOUND ( 'NONE', #11904, .T. ) ;
#18539=CARTESIAN_POINT ( 'NONE',  ( 232.4999999999996305, 83.06687458711267880, -36.86484227207694175 ) ) ;
#18540=EDGE_CURVE ( 'NONE', #17607, #27590, #21084, .T. ) ;
#18549=DIRECTION ( 'NONE',  ( -0.3897722486529259234, 0.9209112846414913012, 1.118268497331688440E-16 ) ) ;
#18573=VECTOR ( 'NONE', #17768, 1000.000000000000000 ) ;
#18584=CARTESIAN_POINT ( 'NONE',  ( 367.4999999999996021, -5.589247009368136787, -100.0000000000000142 ) ) ;
#18612=AXIS2_PLACEMENT_3D ( 'NONE', #11216, #17957, #17524 ) ;
#18643=ADVANCED_FACE ( 'NONE', ( #17201, #6145 ), #10315, .F. ) ;
#18664=ORIENTED_EDGE ( 'NONE', *, *, #21978, .F. ) ;
#18668=VERTEX_POINT ( 'NONE', #6280 ) ;
#18674=DIRECTION ( 'NONE',  ( 1.000000000000000000, -0.000000000000000000, -0.000000000000000000 ) ) ;
#18694=ORIENTED_EDGE ( 'NONE', *, *, #17384, .F. ) ;
#18707=DIRECTION ( 'NONE',  ( 0.000000000000000000, 0.000000000000000000, -1.000000000000000000 ) ) ;
#18708=ORIENTED_EDGE ( 'NONE', *, *, #12971, .T. ) ;
#18812=DIRECTION ( 'NONE',  ( 1.000000000000000000, -0.000000000000000000, -0.000000000000000000 ) ) ;
#18844=ORIENTED_EDGE ( 'NONE', *, *, #22426, .F. ) ;
#18878=CARTESIAN_POINT ( 'NONE',  ( 282.4999999999996589, 19.41075299063184900, 87.99671038392668265 ) ) ;
#18898=DIRECTION ( 'NONE',  ( 1.000000000000000000, 0.000000000000000000, 0.000000000000000000 ) ) ;
#18899=ORIENTED_EDGE ( 'NONE', *, *, #26457, .F. ) ;
#18935=CARTESIAN_POINT ( 'NONE',  ( 217.4999999999996305, 83.06687458711267880, 30.86484227207694886 ) ) ;
#18937=CIRCLE ( 'NONE', #14354, 5.999999999999977796 ) ;
#18950=ADVANCED_FACE ( 'NONE', ( #14457 ), #25221, .F. ) ;
#18955=FACE_OUTER_BOUND ( 'NONE', #21093, .T. ) ;
#18972=PRODUCT ( 'Drill Stand and Mount', 'Drill Stand and Mount', '', ( #11824 ) ) ;
#19032=VECTOR ( 'NONE', #6733, 1000.000000000000000 ) ;
#19037=VECTOR ( 'NONE', #1484, 1000.000000000000000 ) ;
#19140=DIRECTION ( 'NONE',  ( -0.000000000000000000, 0.000000000000000000, 1.000000000000000000 ) ) ;
#19192=CIRCLE ( 'NONE', #7720, 100.0000000000000284 ) ;
#19193=EDGE_LOOP ( 'NONE', ( #19234, #25546, #22759, #11362 ) ) ;
#19234=ORIENTED_EDGE ( 'NONE', *, *, #11548, .F. ) ;
#19236=AXIS2_PLACEMENT_3D ( 'NONE', #7488, #18812, #11670 ) ;
#19284=FACE_BOUND ( 'NONE', #25309, .T. ) ;
#19286=DIRECTION ( 'NONE',  ( -0.000000000000000000, -0.000000000000000000, -1.000000000000000000 ) ) ;
#19289=AXIS2_PLACEMENT_3D ( 'NONE', #8655, #23882, #4332 ) ;
#19370=AXIS2_PLACEMENT_3D ( 'NONE', #2438, #19690, #15106 ) ;
#19379=DIRECTION ( 'NONE',  ( 1.000000000000000000, -0.000000000000000000, -0.000000000000000000 ) ) ;
#19388=VECTOR ( 'NONE', #10258, 1000.000000000000000 ) ;
#19391=DIRECTION ( 'NONE',  ( -1.000000000000000000, 0.000000000000000000, -0.000000000000000000 ) ) ;
#19401=VERTEX_POINT ( 'NONE', #14284 ) ;
#19433=CARTESIAN_POINT ( 'NONE',  ( 372.9108539694884144, -5.589247009368149222, 1.243177022048955014E-14 ) ) ;
#19443=ORIENTED_EDGE ( 'NONE', *, *, #21543, .T. ) ;
#19450=ORIENTED_EDGE ( 'NONE', *, *, #7641, .F. ) ;
#19493=VECTOR ( 'NONE', #6642, 1000.000000000000000 ) ;
#19519=ADVANCED_FACE ( 'NONE', ( #21155 ), #21011, .F. ) ;
#19522=ORIENTED_EDGE ( 'NONE', *, *, #2701, .T. ) ;
#19529=EDGE_CURVE ( 'NONE', #23612, #16763, #12936, .T. ) ;
#19568=DIRECTION ( 'NONE',  ( 1.000000000000000000, -0.000000000000000000, -0.000000000000000000 ) ) ;
#19571=FACE_OUTER_BOUND ( 'NONE', #6888, .T. ) ;
#19587=DIRECTION ( 'NONE',  ( 0.7071067811865474617, 8.659560562354932858E-17, 0.7071067811865474617 ) ) ;
#19610=CARTESIAN_POINT ( 'NONE',  ( 282.4999999999996589, 19.41075299063184900, 87.99671038392668265 ) ) ;
#19613=( NAMED_UNIT ( * ) SI_UNIT ( $, .STERADIAN. ) SOLID_ANGLE_UNIT ( ) );
#19624=VERTEX_POINT ( 'NONE', #19707 ) ;
#19675=CARTESIAN_POINT ( 'NONE',  ( 232.4999999999996305, 83.06687458711267880, 42.86484227207692754 ) ) ;
#19685=PLANE ( 'NONE',  #18612 ) ;
#19690=DIRECTION ( 'NONE',  ( 0.000000000000000000, -1.214306433183764966E-16, 1.000000000000000000 ) ) ;
#19705=EDGE_CURVE ( 'NONE', #12605, #4176, #20278, .T. ) ;
#19707=CARTESIAN_POINT ( 'NONE',  ( 330.9869376377542949, 44.41075299063184190, 75.35061095560295996 ) ) ;
#19708=DIRECTION ( 'NONE',  ( 0.000000000000000000, -1.000000000000000000, -1.214306433183764966E-16 ) ) ;
#19715=ORIENTED_EDGE ( 'NONE', *, *, #4736, .F. ) ;
#19729=CIRCLE ( 'NONE', #12859, 5.999999999999977796 ) ;
#19732=DIRECTION ( 'NONE',  ( 1.000000000000000000, -0.000000000000000000, -0.000000000000000000 ) ) ;
#19743=DIRECTION ( 'NONE',  ( 0.000000000000000000, 0.000000000000000000, -1.000000000000000000 ) ) ;
#19748=LINE ( 'NONE', #25930, #23929 ) ;
#19760=CONICAL_SURFACE ( 'NONE', #19289, 6.025000000000002132, 0.7853981633971707232 ) ;
#19763=ORIENTED_EDGE ( 'NONE', *, *, #3549, .T. ) ;
#19772=LINE ( 'NONE', #15484, #28268 ) ;
#19775=FACE_OUTER_BOUND ( 'NONE', #10086, .T. ) ;
#19796=ORIENTED_EDGE ( 'NONE', *, *, #23003, .T. ) ;
#19801=LINE ( 'NONE', #21822, #13279 ) ;
#19809=CYLINDRICAL_SURFACE ( 'NONE', #21919, 5.999999999999977796 ) ;
#19826=ORIENTED_EDGE ( 'NONE', *, *, #9716, .T. ) ;
#19828=DIRECTION ( 'NONE',  ( 0.000000000000000000, 0.000000000000000000, 1.000000000000000000 ) ) ;
#19846=DIRECTION ( 'NONE',  ( 1.000000000000000000, -0.000000000000000000, -0.000000000000000000 ) ) ;
#19848=CARTESIAN_POINT ( 'NONE',  ( 330.9869376377542949, 44.41075299063183479, -100.0000000000000284 ) ) ;
#19948=DIRECTION ( 'NONE',  ( -9.251858538542974046E-17, -1.214306433183764966E-16, 1.000000000000000000 ) ) ;
#19949=CARTESIAN_POINT ( 'NONE',  ( 367.4999999999996021, 44.41075299063186321, -100.0000000000000142 ) ) ;
#19951=VECTOR ( 'NONE', #15338, 1000.000000000000000 ) ;
#19971=FACE_OUTER_BOUND ( 'NONE', #25374, .T. ) ;
#20015=VECTOR ( 'NONE', #15624, 1000.000000000000114 ) ;
#20048=LINE ( 'NONE', #381, #19951 ) ;
#20064=LINE ( 'NONE', #396, #16074 ) ;
#20091=CARTESIAN_POINT ( 'NONE',  ( 217.4999999999996589, 194.4107529906318064, 100.0000000000000284 ) ) ;
#20092=CIRCLE ( 'NONE', #4026, 5.999999999999991118 ) ;
#20096=FACE_BOUND ( 'NONE', #9684, .T. ) ;
#20147=EDGE_CURVE ( 'NONE', #506, #8492, #18242, .T. ) ;
#20155=ORIENTED_EDGE ( 'NONE', *, *, #14592, .F. ) ;
#20178=VERTEX_POINT ( 'NONE', #9340 ) ;
#20190=ORIENTED_EDGE ( 'NONE', *, *, #12231, .F. ) ;
#20207=DIRECTION ( 'NONE',  ( -1.000000000000000000, 0.000000000000000000, -0.000000000000000000 ) ) ;
#20209=LINE ( 'NONE', #25466, #26618 ) ;
#20252=EDGE_LOOP ( 'NONE', ( #13446, #545, #6706, #9350, #17665, #6443 ) ) ;
#20260=DIRECTION ( 'NONE',  ( 0.000000000000000000, 0.000000000000000000, -1.000000000000000000 ) ) ;
#20270=VECTOR ( 'NONE', #7649, 1000.000000000000114 ) ;
#20272=( GEOMETRIC_REPRESENTATION_CONTEXT ( 3 ) GLOBAL_UNCERTAINTY_ASSIGNED_CONTEXT ( ( #4566 ) ) GLOBAL_UNIT_ASSIGNED_CONTEXT ( ( #22156, #22590, #24601 ) ) REPRESENTATION_CONTEXT ( 'NONE', 'WORKASPACE' ) );
#20278=LINE ( 'NONE', #463, #1923 ) ;
#20285=DIRECTION ( 'NONE',  ( 0.000000000000000000, 0.000000000000000000, -1.000000000000000000 ) ) ;
#20286=ORIENTED_EDGE ( 'NONE', *, *, #7063, .F. ) ;
#20293=ORIENTED_EDGE ( 'NONE', *, *, #14715, .T. ) ;
#20309=CARTESIAN_POINT ( 'NONE',  ( 282.4999999999996589, 19.41075299063184900, 80.49671038392669686 ) ) ;
#20329=LINE ( 'NONE', #9128, #10359 ) ;
#20335=CIRCLE ( 'NONE', #5647, 6.025000000000002132 ) ;
#20338=VECTOR ( 'NONE', #18898, 1000.000000000000000 ) ;
#20345=DIRECTION ( 'NONE',  ( 1.000000000000000000, -0.000000000000000000, -0.000000000000000000 ) ) ;
#20462=CARTESIAN_POINT ( 'NONE',  ( 282.4999999999996589, 19.41075299063184900, 80.49671038392669686 ) ) ;
#20468=CARTESIAN_POINT ( 'NONE',  ( 232.4999999999996305, 133.0668745871126930, -30.86484227207697018 ) ) ;
#20511=AXIS2_PLACEMENT_3D ( 'NONE', #23128, #1283, #14236 ) ;
#20538=EDGE_CURVE ( 'NONE', #7480, #19401, #20335, .T. ) ;
#20572=VERTEX_POINT ( 'NONE', #11577 ) ;
#20612=VERTEX_POINT ( 'NONE', #27336 ) ;
#20628=DIRECTION ( 'NONE',  ( -0.000000000000000000, -0.000000000000000000, -1.000000000000000000 ) ) ;
#20637=DIRECTION ( 'NONE',  ( 0.000000000000000000, -1.000000000000000000, -1.214306433183764966E-16 ) ) ;
#20659=LINE ( 'NONE', #13939, #18186 ) ;
#20694=LINE ( 'NONE', #21117, #13836 ) ;
#20706=EDGE_LOOP ( 'NONE', ( #18694, #25730, #2868, #6229 ) ) ;
#20732=DIRECTION ( 'NONE',  ( 1.000000000000000000, -0.000000000000000000, -0.000000000000000000 ) ) ;
#20745=( GEOMETRIC_REPRESENTATION_CONTEXT ( 3 ) GLOBAL_UNCERTAINTY_ASSIGNED_CONTEXT ( ( #6591 ) ) GLOBAL_UNIT_ASSIGNED_CONTEXT ( ( #17884, #2080, #19613 ) ) REPRESENTATION_CONTEXT ( 'NONE', 'WORKASPACE' ) );
#20786=CIRCLE ( 'NONE', #10700, 5.999999999999991118 ) ;
#20838=DIRECTION ( 'NONE',  ( -0.000000000000000000, -4.625929269271485914E-16, 1.000000000000000000 ) ) ;
#20841=CIRCLE ( 'NONE', #24501, 5.999999999999991118 ) ;
#20899=ORIENTED_EDGE ( 'NONE', *, *, #13450, .F. ) ;
#20911=CARTESIAN_POINT ( 'NONE',  ( 367.4999999999996021, 44.41075299063184900, 1.850330238640837654E-14 ) ) ;
#20948=CARTESIAN_POINT ( 'NONE',  ( 432.4999999999996589, -5.589247009368160768, 100.0000000000000426 ) ) ;
#20961=AXIS2_PLACEMENT_3D ( 'NONE', #18878, #23473, #3787 ) ;
#20968=FACE_OUTER_BOUND ( 'NONE', #13992, .T. ) ;
#20975=DIRECTION ( 'NONE',  ( 1.000000000000000000, -0.000000000000000000, 0.000000000000000000 ) ) ;
#21011=CYLINDRICAL_SURFACE ( 'NONE', #6050, 7.499999999999992895 ) ;
#21026=DIRECTION ( 'NONE',  ( 0.000000000000000000, 1.000000000000000000, 1.214306433183764966E-16 ) ) ;
#21043=CARTESIAN_POINT ( 'NONE',  ( 232.4999999999996305, 133.0668745871126930, -36.86484227207694886 ) ) ;
#21054=ADVANCED_FACE ( 'NONE', ( #27299 ), #24745, .F. ) ;
#21084=LINE ( 'NONE', #24980, #9699 ) ;
#21093=EDGE_LOOP ( 'NONE', ( #10357, #13003, #10643, #8770 ) ) ;
#21117=CARTESIAN_POINT ( 'NONE',  ( 372.9108539694884144, 44.41075299063183479, 167.7200181511720416 ) ) ;
#21128=AXIS2_PLACEMENT_3D ( 'NONE', #13621, #17630, #24524 ) ;
#21135=DIRECTION ( 'NONE',  ( 0.000000000000000000, 0.000000000000000000, 1.000000000000000000 ) ) ;
#21155=FACE_OUTER_BOUND ( 'NONE', #22624, .T. ) ;
#21157=ORIENTED_EDGE ( 'NONE', *, *, #7641, .T. ) ;
#21176=ORIENTED_EDGE ( 'NONE', *, *, #21439, .F. ) ;
#21184=DIRECTION ( 'NONE',  ( -1.000000000000000000, 0.000000000000000000, -0.000000000000000000 ) ) ;
#21201=CARTESIAN_POINT ( 'NONE',  ( 232.4999999999996305, 194.4107529906318064, -75.35061095560291733 ) ) ;
#21209=APPLICATION_CONTEXT ( 'automotive_design' ) ;
#21226=DIRECTION ( 'NONE',  ( -1.000000000000000000, 0.000000000000000000, 0.000000000000000000 ) ) ;
#21227=CARTESIAN_POINT ( 'NONE',  ( 222.4999999999996021, 194.4107529906318064, 58.31593845887894645 ) ) ;
#21229=VERTEX_POINT ( 'NONE', #11404 ) ;
#21245=VERTEX_POINT ( 'NONE', #8953 ) ;
#21255=FACE_BOUND ( 'NONE', #23010, .T. ) ;
#21258=LINE ( 'NONE', #27567, #10944 ) ;
#21260=CARTESIAN_POINT ( 'NONE',  ( 367.4999999999996021, -5.589247009368149222, 1.243177022048955014E-14 ) ) ;
#21372=ORIENTED_EDGE ( 'NONE', *, *, #15203, .F. ) ;
#21379=EDGE_LOOP ( 'NONE', ( #5895, #23861 ) ) ;
#21383=ADVANCED_FACE ( 'NONE', ( #22742 ), #27041, .F. ) ;
#21415=ADVANCED_FACE ( 'NONE', ( #1734 ), #21680, .F. ) ;
#21419=EDGE_CURVE ( 'NONE', #25738, #9830, #5769, .T. ) ;
#21426=LINE ( 'NONE', #8504, #10241 ) ;
#21434=DIRECTION ( 'NONE',  ( 0.000000000000000000, 0.000000000000000000, -1.000000000000000000 ) ) ;
#21435=CARTESIAN_POINT ( 'NONE',  ( 267.4999999999996021, 194.4107529906318064, 288.0938197134494203 ) ) ;
#21439=EDGE_CURVE ( 'NONE', #2977, #12526, #18937, .T. ) ;
#21460=DIRECTION ( 'NONE',  ( 1.000000000000000000, -0.000000000000000000, -0.000000000000000000 ) ) ;
#21478=CYLINDRICAL_SURFACE ( 'NONE', #23145, 5.999999999999977796 ) ;
#21479=DIRECTION ( 'NONE',  ( 0.7071067811867438602, 0.000000000000000000, -0.7071067811863512853 ) ) ;
#21484=ORIENTED_EDGE ( 'NONE', *, *, #14714, .T. ) ;
#21540=ADVANCED_FACE ( 'NONE', ( #15798 ), #22533, .F. ) ;
#21543=EDGE_CURVE ( 'NONE', #27217, #18668, #2697, .T. ) ;
#21554=ORIENTED_EDGE ( 'NONE', *, *, #26457, .T. ) ;
#21562=DIRECTION ( 'NONE',  ( 0.000000000000000000, 0.000000000000000000, -1.000000000000000000 ) ) ;
#21563=CARTESIAN_POINT ( 'NONE',  ( 232.4999999999996305, 194.4107529906318348, 58.31593845887914540 ) ) ;
#21580=CARTESIAN_POINT ( 'NONE',  ( 367.4999999999996021, 44.41075299063184900, 1.850330238640837654E-14 ) ) ;
#21610=ORIENTED_EDGE ( 'NONE', *, *, #16939, .T. ) ;
#21628=LINE ( 'NONE', #7996, #25829 ) ;
#21670=ORIENTED_EDGE ( 'NONE', *, *, #23739, .T. ) ;
#21674=EDGE_CURVE ( 'NONE', #21229, #20572, #24431, .T. ) ;
#21680=CONICAL_SURFACE ( 'NONE', #25352, 6.025000000000002132, 0.7853981633971707232 ) ;
#21684=CARTESIAN_POINT ( 'NONE',  ( 217.4999999999996305, -5.589247009368136787, -100.0000000000000142 ) ) ;
#21691=EDGE_CURVE ( 'NONE', #15333, #21229, #14483, .T. ) ;
#21704=PLANE ( 'NONE',  #19370 ) ;
#21757=CARTESIAN_POINT ( 'NONE',  ( 222.4999999999996021, 194.4107529906318064, -62.90796922943941638 ) ) ;
#21813=EDGE_LOOP ( 'NONE', ( #19450, #15473 ) ) ;
#21822=CARTESIAN_POINT ( 'NONE',  ( 367.4999999999996021, -5.589247009368160768, 100.0000000000000284 ) ) ;
#21873=ORIENTED_EDGE ( 'NONE', *, *, #21674, .F. ) ;
#21878=ORIENTED_EDGE ( 'NONE', *, *, #22454, .F. ) ;
#21899=LINE ( 'NONE', #6673, #1990 ) ;
#21901=ORIENTED_EDGE ( 'NONE', *, *, #22423, .F. ) ;
#21908=LINE ( 'NONE', #17028, #27947 ) ;
#21919=AXIS2_PLACEMENT_3D ( 'NONE', #11922, #22545, #9618 ) ;
#21938=AXIS2_PLACEMENT_3D ( 'NONE', #4266, #10747, #23815 ) ;
#21942=FACE_OUTER_BOUND ( 'NONE', #16962, .T. ) ;
#21946=ORIENTED_EDGE ( 'NONE', *, *, #15631, .F. ) ;
#21949=ORIENTED_EDGE ( 'NONE', *, *, #16816, .F. ) ;
#21970=CARTESIAN_POINT ( 'NONE',  ( 372.9108539694884144, 44.41075299063183479, 100.0000000000000284 ) ) ;
#21974=LINE ( 'NONE', #26287, #27941 ) ;
#21978=EDGE_CURVE ( 'NONE', #15680, #9277, #14584, .T. ) ;
#21991=CONICAL_SURFACE ( 'NONE', #431, 6.025000000000002132, 0.7853981633971707232 ) ;
#21998=AXIS2_PLACEMENT_3D ( 'NONE', #18539, #18674, #14098 ) ;
#22013=SHAPE_REPRESENTATION ( 'Drill Stand and Mount', ( #10637 ), #20272 ) ;
#22035=CIRCLE ( 'NONE', #7812, 6.025000000000002132 ) ;
#22098=CARTESIAN_POINT ( 'NONE',  ( 367.9108539694884144, -5.589247009368160768, 100.0000000000000284 ) ) ;
#22103=CARTESIAN_POINT ( 'NONE',  ( 232.4749999999995964, 133.0668745871126930, 36.86484227207694886 ) ) ;
#22111=FACE_BOUND ( 'NONE', #24993, .T. ) ;
#22115=CARTESIAN_POINT ( 'NONE',  ( 372.9108539694884144, 44.41075299063183479, 100.0000000000000284 ) ) ;
#22156=( LENGTH_UNIT ( ) NAMED_UNIT ( * ) SI_UNIT ( .MILLI., .METRE. ) );
#22158=AXIS2_PLACEMENT_3D ( 'NONE', #260, #7149, #15928 ) ;
#22252=CARTESIAN_POINT ( 'NONE',  ( 232.4999999999996305, 83.06687458711267880, 36.86484227207694175 ) ) ;
#22291=DIRECTION ( 'NONE',  ( -1.000000000000000000, 0.000000000000000000, 0.000000000000000000 ) ) ;
#22339=DIRECTION ( 'NONE',  ( -0.000000000000000000, -0.3247168404252948060, -0.9458112779747414045 ) ) ;
#22373=ORIENTED_EDGE ( 'NONE', *, *, #25090, .T. ) ;
#22380=VERTEX_POINT ( 'NONE', #3473 ) ;
#22410=CARTESIAN_POINT ( 'NONE',  ( 232.4749999999995964, 133.0668745871126930, -36.86484227207694886 ) ) ;
#22423=EDGE_CURVE ( 'NONE', #27590, #26144, #21426, .T. ) ;
#22426=EDGE_CURVE ( 'NONE', #24580, #16161, #26291, .T. ) ;
#22432=AXIS2_PLACEMENT_3D ( 'NONE', #15311, #8554, #14886 ) ;
#22454=EDGE_CURVE ( 'NONE', #23614, #27147, #25731, .T. ) ;
#22493=ORIENTED_EDGE ( 'NONE', *, *, #23878, .F. ) ;
#22533=PLANE ( 'NONE',  #2876 ) ;
#22539=DIRECTION ( 'NONE',  ( 0.000000000000000000, -1.000000000000000000, -1.214306433183764966E-16 ) ) ;
#22545=DIRECTION ( 'NONE',  ( 1.000000000000000000, -0.000000000000000000, -0.000000000000000000 ) ) ;
#22546=DIRECTION ( 'NONE',  ( 0.000000000000000000, 0.000000000000000000, -1.000000000000000000 ) ) ;
#22585=ORIENTED_EDGE ( 'NONE', *, *, #5559, .T. ) ;
#22586=CARTESIAN_POINT ( 'NONE',  ( 267.4999999999996021, 194.4107529906318064, 288.0938197134494203 ) ) ;
#22587=DIRECTION ( 'NONE',  ( 0.000000000000000000, 9.251858538542967883E-17, -1.000000000000000000 ) ) ;
#22590=( NAMED_UNIT ( * ) PLANE_ANGLE_UNIT ( ) SI_UNIT ( $, .RADIAN. ) );
#22600=CIRCLE ( 'NONE', #8386, 5.999999999999977796 ) ;
#22613=AXIS2_PLACEMENT_3D ( 'NONE', #2983, #12051, #3115 ) ;
#22624=EDGE_LOOP ( 'NONE', ( #18327, #9260, #14094, #8249 ) ) ;
#22686=CARTESIAN_POINT ( 'NONE',  ( 367.4999999999996021, 44.41075299063183479, 100.0000000000000284 ) ) ;
#22727=ORIENTED_EDGE ( 'NONE', *, *, #20538, .F. ) ;
#22742=FACE_OUTER_BOUND ( 'NONE', #915, .T. ) ;
#22753=CARTESIAN_POINT ( 'NONE',  ( 372.9108539694884144, 19.41075299063184900, 87.99671038392668265 ) ) ;
#22759=ORIENTED_EDGE ( 'NONE', *, *, #21419, .T. ) ;
#22800=AXIS2_PLACEMENT_3D ( 'NONE', #13890, #2657, #7410 ) ;
#22806=EDGE_LOOP ( 'NONE', ( #11546, #3849, #19522, #4286 ) ) ;
#22824=DIRECTION ( 'NONE',  ( 0.000000000000000000, 1.272130549049657961E-16, -1.000000000000000000 ) ) ;
#22849=CYLINDRICAL_SURFACE ( 'NONE', #19236, 5.999999999999991118 ) ;
#22866=ORIENTED_EDGE ( 'NONE', *, *, #6941, .F. ) ;
#22873=ORIENTED_EDGE ( 'NONE', *, *, #10889, .F. ) ;
#22928=DIRECTION ( 'NONE',  ( 0.000000000000000000, 0.000000000000000000, -1.000000000000000000 ) ) ;
#22943=ORIENTED_EDGE ( 'NONE', *, *, #14697, .T. ) ;
#22957=LINE ( 'NONE', #24545, #16261 ) ;
#22987=CARTESIAN_POINT ( 'NONE',  ( 267.4999999999996021, 194.4107529906318064, 100.0000000000000284 ) ) ;
#23003=EDGE_CURVE ( 'NONE', #9740, #24079, #2269, .T. ) ;
#23010=EDGE_LOOP ( 'NONE', ( #4810, #12801 ) ) ;
#23025=CARTESIAN_POINT ( 'NONE',  ( 232.4999999999996305, 83.06687458711267880, -42.88984227207694033 ) ) ;
#23057=EDGE_CURVE ( 'NONE', #19401, #7480, #9813, .T. ) ;
#23118=ORIENTED_EDGE ( 'NONE', *, *, #9436, .F. ) ;
#23123=VERTEX_POINT ( 'NONE', #15804 ) ;
#23128=CARTESIAN_POINT ( 'NONE',  ( 217.4999999999996305, 133.0668745871126930, -36.86484227207694886 ) ) ;
#23135=DIRECTION ( 'NONE',  ( -1.000000000000000000, 0.000000000000000000, -0.000000000000000000 ) ) ;
#23145=AXIS2_PLACEMENT_3D ( 'NONE', #8417, #3813, #13025 ) ;
#23166=EDGE_CURVE ( 'NONE', #26679, #19624, #22957, .T. ) ;
#23178=DIRECTION ( 'NONE',  ( 1.000000000000000000, -0.000000000000000000, -0.000000000000000000 ) ) ;
#23227=ORIENTED_EDGE ( 'NONE', *, *, #7865, .F. ) ;
#23242=CIRCLE ( 'NONE', #22800, 5.999999999999977796 ) ;
#23268=ADVANCED_FACE ( 'NONE', ( #15013 ), #23764, .F. ) ;
#23324=ORIENTED_EDGE ( 'NONE', *, *, #26791, .F. ) ;
#23345=LINE ( 'NONE', #10415, #25712 ) ;
#23461=DIRECTION ( 'NONE',  ( 0.000000000000000000, -1.214306433183764966E-16, 1.000000000000000000 ) ) ;
#23473=DIRECTION ( 'NONE',  ( 1.000000000000000000, -0.000000000000000000, -0.000000000000000000 ) ) ;
#23487=VERTEX_POINT ( 'NONE', #14136 ) ;
#23528=LINE ( 'NONE', #21227, #18259 ) ;
#23539=ORIENTED_EDGE ( 'NONE', *, *, #16395, .T. ) ;
#23547=ORIENTED_EDGE ( 'NONE', *, *, #24177, .T. ) ;
#23548=VERTEX_POINT ( 'NONE', #23025 ) ;
#23598=CARTESIAN_POINT ( 'NONE',  ( 232.4749999999995964, 83.06687458711267880, -36.86484227207694175 ) ) ;
#23606=VERTEX_POINT ( 'NONE', #12826 ) ;
#23612=VERTEX_POINT ( 'NONE', #14690 ) ;
#23614=VERTEX_POINT ( 'NONE', #26017 ) ;
#23680=VECTOR ( 'NONE', #17506, 1000.000000000000000 ) ;
#23682=ORIENTED_EDGE ( 'NONE', *, *, #23878, .T. ) ;
#23697=AXIS2_PLACEMENT_3D ( 'NONE', #24369, #17907, #13613 ) ;
#23715=ADVANCED_FACE ( 'NONE', ( #4325 ), #8783, .F. ) ;
#23732=DIRECTION ( 'NONE',  ( 1.000000000000000000, -0.000000000000000000, -0.000000000000000000 ) ) ;
#23735=FACE_OUTER_BOUND ( 'NONE', #10793, .T. ) ;
#23739=EDGE_CURVE ( 'NONE', #9830, #25647, #15840, .T. ) ;
#23757=VERTEX_POINT ( 'NONE', #17688 ) ;
#23764=CYLINDRICAL_SURFACE ( 'NONE', #24968, 5.999999999999977796 ) ;
#23766=CARTESIAN_POINT ( 'NONE',  ( 232.4999999999996305, 194.4107529906318064, -62.90796922943941638 ) ) ;
#23815=DIRECTION ( 'NONE',  ( 0.000000000000000000, 0.000000000000000000, -1.000000000000000000 ) ) ;
#23861=ORIENTED_EDGE ( 'NONE', *, *, #2826, .F. ) ;
#23869=DIRECTION ( 'NONE',  ( 0.000000000000000000, -0.3247168404252948615, -0.9458112779747414045 ) ) ;
#23878=EDGE_CURVE ( 'NONE', #26636, #23123, #17212, .T. ) ;
#23882=DIRECTION ( 'NONE',  ( 1.000000000000000000, -0.000000000000000000, -0.000000000000000000 ) ) ;
#23929=VECTOR ( 'NONE', #21479, 1000.000000000000114 ) ;
#23940=ORIENTED_EDGE ( 'NONE', *, *, #11340, .T. ) ;
#23984=DIRECTION ( 'NONE',  ( 0.3897722486529259234, -0.9209112846414911902, 0.000000000000000000 ) ) ;
#24042=ORIENTED_EDGE ( 'NONE', *, *, #743, .T. ) ;
#24079=VERTEX_POINT ( 'NONE', #10341 ) ;
#24112=EDGE_CURVE ( 'NONE', #15680, #5949, #10626, .T. ) ;
#24124=CIRCLE ( 'NONE', #18159, 5.999999999999991118 ) ;
#24129=CARTESIAN_POINT ( 'NONE',  ( 232.4999999999996305, 133.0668745871126930, -36.86484227207694886 ) ) ;
#24155=CIRCLE ( 'NONE', #23697, 5.999999999999977796 ) ;
#24170=CARTESIAN_POINT ( 'NONE',  ( 367.4999999999996021, 44.41075299063184900, 1.850330238640837654E-14 ) ) ;
#24177=EDGE_CURVE ( 'NONE', #5808, #12260, #2276, .T. ) ;
#24191=DIRECTION ( 'NONE',  ( 0.000000000000000000, 0.000000000000000000, -1.000000000000000000 ) ) ;
#24199=CARTESIAN_POINT ( 'NONE',  ( 267.4999999999996021, 194.4107529906318064, -75.35061095560291733 ) ) ;
#24221=ORIENTED_EDGE ( 'NONE', *, *, #27794, .T. ) ;
#24256=AXIS2_PLACEMENT_3D ( 'NONE', #22753, #11843, #9680 ) ;
#24369=CARTESIAN_POINT ( 'NONE',  ( 217.4999999999996305, 133.0668745871126930, 36.86484227207694886 ) ) ;
#24431=CIRCLE ( 'NONE', #22613, 7.499999999999992895 ) ;
#24450=VERTEX_POINT ( 'NONE', #12905 ) ;
#24485=DIRECTION ( 'NONE',  ( -0.000000000000000000, -0.000000000000000000, -1.000000000000000000 ) ) ;
#24501=AXIS2_PLACEMENT_3D ( 'NONE', #5044, #3165, #11954 ) ;
#24513=AXIS2_PLACEMENT_3D ( 'NONE', #15545, #17977, #2739 ) ;
#24524=DIRECTION ( 'NONE',  ( 0.000000000000000000, 9.251858538542967883E-17, -1.000000000000000000 ) ) ;
#24545=CARTESIAN_POINT ( 'NONE',  ( 267.4999999999996021, 194.4107529906318348, 75.35061095560300259 ) ) ;
#24571=DIRECTION ( 'NONE',  ( 0.7071067811867438602, 8.659560562352529298E-17, 0.7071067811863512853 ) ) ;
#24580=VERTEX_POINT ( 'NONE', #15485 ) ;
#24601=( NAMED_UNIT ( * ) SI_UNIT ( $, .STERADIAN. ) SOLID_ANGLE_UNIT ( ) );
#24607=ORIENTED_EDGE ( 'NONE', *, *, #7624, .T. ) ;
#24621=LINE ( 'NONE', #16013, #8196 ) ;
#24686=DIRECTION ( 'NONE',  ( 0.000000000000000000, 1.214306433183764966E-16, -1.000000000000000000 ) ) ;
#24692=FACE_OUTER_BOUND ( 'NONE', #2020, .T. ) ;
#24704=FACE_OUTER_BOUND ( 'NONE', #12498, .T. ) ;
#24706=CARTESIAN_POINT ( 'NONE',  ( 232.4999999999996305, 194.4107529906318064, 288.0938197134494203 ) ) ;
#24715=LINE ( 'NONE', #7046, #117 ) ;
#24718=CIRCLE ( 'NONE', #24256, 7.499999999999992895 ) ;
#24729=DIRECTION ( 'NONE',  ( 0.000000000000000000, 9.251858538542967883E-17, -1.000000000000000000 ) ) ;
#24745=CYLINDRICAL_SURFACE ( 'NONE', #9351, 75.00000000000002842 ) ;
#24809=CARTESIAN_POINT ( 'NONE',  ( 217.4999999999996305, 83.06687458711267880, 36.86484227207694175 ) ) ;
#24824=ORIENTED_EDGE ( 'NONE', *, *, #4702, .T. ) ;
#24826=ORIENTED_EDGE ( 'NONE', *, *, #1064, .T. ) ;
#24828=ORIENTED_EDGE ( 'NONE', *, *, #13450, .T. ) ;
#24831=CARTESIAN_POINT ( 'NONE',  ( 367.9108539694884144, -5.589247009368149222, 1.243177022048955014E-14 ) ) ;
#24832=AXIS2_PLACEMENT_3D ( 'NONE', #2033, #23732, #10663 ) ;
#24842=DIRECTION ( 'NONE',  ( 1.000000000000000000, -0.000000000000000000, -0.000000000000000000 ) ) ;
#24926=FACE_OUTER_BOUND ( 'NONE', #12816, .T. ) ;
#24944=DIRECTION ( 'NONE',  ( 1.000000000000000000, 0.000000000000000000, 0.000000000000000000 ) ) ;
#24962=EDGE_LOOP ( 'NONE', ( #21176, #15431 ) ) ;
#24968=AXIS2_PLACEMENT_3D ( 'NONE', #4075, #10837, #12861 ) ;
#24980=CARTESIAN_POINT ( 'NONE',  ( 232.4999999999996305, 133.0668745871126930, 42.86484227207692044 ) ) ;
#24982=CARTESIAN_POINT ( 'NONE',  ( 217.4999999999996305, 194.4107529906318064, -100.0000000000000000 ) ) ;
#24993=EDGE_LOOP ( 'NONE', ( #27571, #22727 ) ) ;
#25065=CARTESIAN_POINT ( 'NONE',  ( 0.000000000000000000, 0.000000000000000000, 0.000000000000000000 ) ) ;
#25075=ORIENTED_EDGE ( 'NONE', *, *, #6294, .T. ) ;
#25082=LINE ( 'NONE', #11883, #16326 ) ;
#25085=DIRECTION ( 'NONE',  ( 0.000000000000000000, 0.000000000000000000, -1.000000000000000000 ) ) ;
#25090=EDGE_CURVE ( 'NONE', #23123, #7575, #20329, .T. ) ;
#25140=ADVANCED_FACE ( 'NONE', ( #3783 ), #16451, .F. ) ;
#25141=DIRECTION ( 'NONE',  ( 0.000000000000000000, -1.000000000000000000, -1.214306433183764966E-16 ) ) ;
#25162=ORIENTED_EDGE ( 'NONE', *, *, #1571, .F. ) ;
#25221=CYLINDRICAL_SURFACE ( 'NONE', #18425, 7.499999999999992895 ) ;
#25231=EDGE_LOOP ( 'NONE', ( #15327, #26532, #23324, #27796 ) ) ;
#25270=ORIENTED_EDGE ( 'NONE', *, *, #2688, .T. ) ;
#25274=VERTEX_POINT ( 'NONE', #7224 ) ;
#25307=CARTESIAN_POINT ( 'NONE',  ( 232.4999999999996305, 83.06687458711267880, 36.86484227207694175 ) ) ;
#25309=EDGE_LOOP ( 'NONE', ( #16694, #146 ) ) ;
#25339=LINE ( 'NONE', #4056, #19388 ) ;
#25345=ORIENTED_EDGE ( 'NONE', *, *, #20147, .T. ) ;
#25352=AXIS2_PLACEMENT_3D ( 'NONE', #25307, #10369, #21562 ) ;
#25357=CARTESIAN_POINT ( 'NONE',  ( 282.4999999999996589, 19.41075299063184900, 87.99671038392668265 ) ) ;
#25363=DIRECTION ( 'NONE',  ( 1.000000000000000000, -0.000000000000000000, -0.000000000000000000 ) ) ;
#25374=EDGE_LOOP ( 'NONE', ( #3216, #3363, #9522, #4130 ) ) ;
#25412=ORIENTED_EDGE ( 'NONE', *, *, #8807, .F. ) ;
#25425=DIRECTION ( 'NONE',  ( -0.000000000000000000, 0.000000000000000000, 1.000000000000000000 ) ) ;
#25449=DIRECTION ( 'NONE',  ( -0.000000000000000000, -1.000000000000000000, -0.000000000000000000 ) ) ;
#25466=CARTESIAN_POINT ( 'NONE',  ( 232.4999999999996305, 133.0668745871126930, -42.86484227207692044 ) ) ;
#25468=CYLINDRICAL_SURFACE ( 'NONE', #13518, 75.00000000000002842 ) ;
#25476=CARTESIAN_POINT ( 'NONE',  ( 217.4999999999996305, -5.589247009368160768, 100.0000000000000142 ) ) ;
#25546=ORIENTED_EDGE ( 'NONE', *, *, #15833, .T. ) ;
#25581=ORIENTED_EDGE ( 'NONE', *, *, #24112, .F. ) ;
#25647=VERTEX_POINT ( 'NONE', #13961 ) ;
#25666=CIRCLE ( 'NONE', #8223, 5.999999999999977796 ) ;
#25695=ORIENTED_EDGE ( 'NONE', *, *, #14168, .F. ) ;
#25708=DIRECTION ( 'NONE',  ( 0.000000000000000000, 0.000000000000000000, 1.000000000000000000 ) ) ;
#25712=VECTOR ( 'NONE', #27782, 1000.000000000000000 ) ;
#25730=ORIENTED_EDGE ( 'NONE', *, *, #26305, .T. ) ;
#25731=LINE ( 'NONE', #28164, #1522 ) ;
#25738=VERTEX_POINT ( 'NONE', #8284 ) ;
#25740=CARTESIAN_POINT ( 'NONE',  ( 367.4999999999996021, -5.589247009368139452, -75.00000000000001421 ) ) ;
#25755=FACE_OUTER_BOUND ( 'NONE', #20252, .T. ) ;
#25771=LINE ( 'NONE', #23766, #7827 ) ;
#25787=DIRECTION ( 'NONE',  ( 1.000000000000000000, 0.000000000000000000, 0.000000000000000000 ) ) ;
#25824=DIRECTION ( 'NONE',  ( 0.000000000000000000, 0.000000000000000000, -1.000000000000000000 ) ) ;
#25829=VECTOR ( 'NONE', #5834, 1000.000000000000000 ) ;
#25928=DIRECTION ( 'NONE',  ( 0.000000000000000000, 0.000000000000000000, -1.000000000000000000 ) ) ;
#25930=CARTESIAN_POINT ( 'NONE',  ( 232.4999999999996305, 83.06687458711267880, -42.88984227207694033 ) ) ;
#25952=EDGE_CURVE ( 'NONE', #27147, #27590, #23242, .T. ) ;
#25974=EDGE_LOOP ( 'NONE', ( #18127, #27659, #17009, #17248 ) ) ;
#25985=DIRECTION ( 'NONE',  ( 1.000000000000000000, -0.000000000000000000, -0.000000000000000000 ) ) ;
#26013=VERTEX_POINT ( 'NONE', #18191 ) ;
#26017=CARTESIAN_POINT ( 'NONE',  ( 217.4999999999996305, 133.0668745871126930, 30.86484227207697018 ) ) ;
#26033=VERTEX_POINT ( 'NONE', #15756 ) ;
#26095=CARTESIAN_POINT ( 'NONE',  ( 432.4999999999996589, 0.000000000000000000, 0.000000000000000000 ) ) ;
#26127=CIRCLE ( 'NONE', #13772, 7.499999999999992895 ) ;
#26136=CARTESIAN_POINT ( 'NONE',  ( 217.4999999999996305, 133.0668745871126930, 36.86484227207694886 ) ) ;
#26141=EDGE_CURVE ( 'NONE', #506, #12924, #14443, .T. ) ;
#26144=VERTEX_POINT ( 'NONE', #27768 ) ;
#26157=ORIENTED_EDGE ( 'NONE', *, *, #9136, .T. ) ;
#26174=ADVANCED_FACE ( 'NONE', ( #7825 ), #5946, .F. ) ;
#26183=ORIENTED_EDGE ( 'NONE', *, *, #17947, .F. ) ;
#26194=CARTESIAN_POINT ( 'NONE',  ( 330.9869376377542949, 44.41075299063185611, -75.35061095560293154 ) ) ;
#26216=EDGE_LOOP ( 'NONE', ( #25270, #18664, #11301, #1251 ) ) ;
#26219=ORIENTED_EDGE ( 'NONE', *, *, #15059, .T. ) ;
#26241=CARTESIAN_POINT ( 'NONE',  ( 367.4999999999996021, 44.41075299063183479, 100.0000000000000284 ) ) ;
#26287=CARTESIAN_POINT ( 'NONE',  ( 372.9108539694884144, 44.41075299063184190, 74.80456309157131045 ) ) ;
#26291=CIRCLE ( 'NONE', #13936, 5.999999999999991118 ) ;
#26305=EDGE_CURVE ( 'NONE', #24450, #17486, #10689, .T. ) ;
#26308=LINE ( 'NONE', #6635, #8667 ) ;
#26317=CARTESIAN_POINT ( 'NONE',  ( 330.9869376377542949, 44.41075299063183479, 288.0938197134494203 ) ) ;
#26330=VECTOR ( 'NONE', #19286, 1000.000000000000000 ) ;
#26383=LINE ( 'NONE', #26825, #17498 ) ;
#26433=ORIENTED_EDGE ( 'NONE', *, *, #18399, .T. ) ;
#26448=CARTESIAN_POINT ( 'NONE',  ( 432.4999999999996589, 19.41075299063184900, 87.99671038392668265 ) ) ;
#26457=EDGE_CURVE ( 'NONE', #5949, #24079, #9239, .T. ) ;
#26471=VERTEX_POINT ( 'NONE', #27866 ) ;
#26529=EDGE_LOOP ( 'NONE', ( #17351, #17886, #6102, #2181 ) ) ;
#26532=ORIENTED_EDGE ( 'NONE', *, *, #12389, .F. ) ;
#26536=CARTESIAN_POINT ( 'NONE',  ( 222.4999999999996021, 186.4134324495536248, 35.02193266779035952 ) ) ;
#26618=VECTOR ( 'NONE', #27607, 1000.000000000000000 ) ;
#26636=VERTEX_POINT ( 'NONE', #11225 ) ;
#26679=VERTEX_POINT ( 'NONE', #3017 ) ;
#26771=EDGE_CURVE ( 'NONE', #12526, #2977, #6742, .T. ) ;
#26782=CARTESIAN_POINT ( 'NONE',  ( 432.4999999999996589, 19.41075299063184900, 87.99671038392668265 ) ) ;
#26791=EDGE_CURVE ( 'NONE', #23606, #20612, #27555, .T. ) ;
#26825=CARTESIAN_POINT ( 'NONE',  ( 267.4999999999996021, 194.4107529906318348, -75.35061095560291733 ) ) ;
#26835=ORIENTED_EDGE ( 'NONE', *, *, #21691, .T. ) ;
#26859=ORIENTED_EDGE ( 'NONE', *, *, #28135, .F. ) ;
#26875=ADVANCED_FACE ( 'NONE', ( #18955 ), #10197, .T. ) ;
#26926=LINE ( 'NONE', #20462, #10063 ) ;
#26955=CARTESIAN_POINT ( 'NONE',  ( 282.4999999999996589, 19.41075299063184900, 87.99671038392668265 ) ) ;
#27027=CONICAL_SURFACE ( 'NONE', #5920, 6.025000000000002132, 0.7853981633974482790 ) ;
#27041=PLANE ( 'NONE',  #5156 ) ;
#27064=ORIENTED_EDGE ( 'NONE', *, *, #1571, .T. ) ;
#27082=EDGE_LOOP ( 'NONE', ( #26183, #3357, #13206, #25345, #25075, #11567, #6481, #19796 ) ) ;
#27131=FACE_BOUND ( 'NONE', #21813, .T. ) ;
#27147=VERTEX_POINT ( 'NONE', #4563 ) ;
#27159=STYLED_ITEM('',(#28434),#8800);
#27200=LINE ( 'NONE', #7537, #1550 ) ;
#27217=VERTEX_POINT ( 'NONE', #22098 ) ;
#27265=DIRECTION ( 'NONE',  ( 1.000000000000000000, -0.000000000000000000, -0.000000000000000000 ) ) ;
#27294=LINE ( 'NONE', #7908, #14279 ) ;
#27299=FACE_OUTER_BOUND ( 'NONE', #6118, .T. ) ;
#27336=CARTESIAN_POINT ( 'NONE',  ( 267.4999999999996021, 194.4107529906318064, 100.0000000000000284 ) ) ;
#27417=AXIS2_PLACEMENT_3D ( 'NONE', #16508, #27265, #7602 ) ;
#27494=FACE_OUTER_BOUND ( 'NONE', #6969, .T. ) ;
#27496=DIRECTION ( 'NONE',  ( 1.000000000000000000, -0.000000000000000000, -0.000000000000000000 ) ) ;
#27497=CIRCLE ( 'NONE', #16072, 6.025000000000002132 ) ;
#27502=FACE_OUTER_BOUND ( 'NONE', #20706, .T. ) ;
#27537=DIRECTION ( 'NONE',  ( 0.000000000000000000, 0.000000000000000000, -1.000000000000000000 ) ) ;
#27555=LINE ( 'NONE', #22987, #11358 ) ;
#27567=CARTESIAN_POINT ( 'NONE',  ( 432.4999999999996589, 44.41075299063184190, 100.0000000000000426 ) ) ;
#27571=ORIENTED_EDGE ( 'NONE', *, *, #23057, .F. ) ;
#27590=VERTEX_POINT ( 'NONE', #6054 ) ;
#27597=CARTESIAN_POINT ( 'NONE',  ( 267.4999999999996021, 194.4107529906318064, 288.0938197134494203 ) ) ;
#27607=DIRECTION ( 'NONE',  ( 1.000000000000000000, -0.000000000000000000, -0.000000000000000000 ) ) ;
#27641=CARTESIAN_POINT ( 'NONE',  ( 217.4999999999996305, 83.06687458711267880, 36.86484227207694175 ) ) ;
#27642=CARTESIAN_POINT ( 'NONE',  ( 282.4999999999996589, 19.41075299063184900, 87.99671038392668265 ) ) ;
#27659=ORIENTED_EDGE ( 'NONE', *, *, #12720, .T. ) ;
#27662=ADVANCED_FACE ( 'NONE', ( #5911 ), #21991, .F. ) ;
#27675=PRODUCT_DEFINITION_SHAPE ( 'NONE', 'NONE',  #18451 ) ;
#27683=ORIENTED_EDGE ( 'NONE', *, *, #11774, .F. ) ;
#27694=ORIENTED_EDGE ( 'NONE', *, *, #26771, .T. ) ;
#27751=DIRECTION ( 'NONE',  ( 0.000000000000000000, 9.251858538542967883E-17, -1.000000000000000000 ) ) ;
#27754=ORIENTED_EDGE ( 'NONE', *, *, #4702, .F. ) ;
#27768=CARTESIAN_POINT ( 'NONE',  ( 232.4999999999996305, 133.0668745871126930, 42.88984227207694744 ) ) ;
#27782=DIRECTION ( 'NONE',  ( 0.000000000000000000, -1.000000000000000000, -1.214306433183764966E-16 ) ) ;
#27794=EDGE_CURVE ( 'NONE', #8019, #9011, #13067, .T. ) ;
#27796=ORIENTED_EDGE ( 'NONE', *, *, #13622, .T. ) ;
#27821=EDGE_CURVE ( 'NONE', #9740, #17744, #4281, .T. ) ;
#27845=AXIS2_PLACEMENT_3D ( 'NONE', #8036, #7623, #10336 ) ;
#27866=CARTESIAN_POINT ( 'NONE',  ( 217.4999999999996305, 83.06687458711267880, -42.86484227207692754 ) ) ;
#27941=VECTOR ( 'NONE', #15389, 1000.000000000000000 ) ;
#27947=VECTOR ( 'NONE', #28072, 1000.000000000000000 ) ;
#27955=LINE ( 'NONE', #12341, #8544 ) ;
#27967=ORIENTED_EDGE ( 'NONE', *, *, #14168, .T. ) ;
#27995=FACE_OUTER_BOUND ( 'NONE', #3082, .T. ) ;
#28005=AXIS2_PLACEMENT_3D ( 'NONE', #6346, #10384, #19140 ) ;
#28014=DIRECTION ( 'NONE',  ( -1.000000000000000000, 0.000000000000000000, -0.000000000000000000 ) ) ;
#28072=DIRECTION ( 'NONE',  ( 1.000000000000000000, -0.000000000000000000, -0.000000000000000000 ) ) ;
#28102=LINE ( 'NONE', #26241, #14621 ) ;
#28104=ORIENTED_EDGE ( 'NONE', *, *, #8999, .T. ) ;
#28106=VECTOR ( 'NONE', #2059, 1000.000000000000000 ) ;
#28130=DIRECTION ( 'NONE',  ( 0.000000000000000000, 0.000000000000000000, -1.000000000000000000 ) ) ;
#28135=EDGE_CURVE ( 'NONE', #23612, #23548, #19748, .T. ) ;
#28136=EDGE_CURVE ( 'NONE', #26013, #12924, #17593, .T. ) ;
#28151=DIRECTION ( 'NONE',  ( -1.000000000000000000, 0.000000000000000000, -0.000000000000000000 ) ) ;
#28163=VECTOR ( 'NONE', #11085, 1000.000000000000000 ) ;
#28164=CARTESIAN_POINT ( 'NONE',  ( 232.4999999999996305, 133.0668745871126930, 30.86484227207697018 ) ) ;
#28236=EDGE_CURVE ( 'NONE', #12526, #24450, #13589, .T. ) ;
#28245=DIRECTION ( 'NONE',  ( -1.000000000000000000, 0.000000000000000000, -9.251858538542972814E-17 ) ) ;
#28252=DIRECTION ( 'NONE',  ( 1.000000000000000000, -0.000000000000000000, -0.000000000000000000 ) ) ;
#28268=VECTOR ( 'NONE', #4263, 1000.000000000000000 ) ;
#28304=CARTESIAN_POINT ( 'NONE',  ( 267.4999999999996021, 194.4107529906318064, 288.0938197134494203 ) ) ;
#28348=CARTESIAN_POINT ( 'NONE',  ( 367.4999999999996021, 44.41075299063186321, -100.0000000000000142 ) ) ;
#28356=CIRCLE ( 'NONE', #7290, 75.00000000000002842 ) ;
#28357=ORIENTED_EDGE ( 'NONE', *, *, #10649, .F. ) ;
#28428=COLOUR_RGB('Sky Blue',0.24,0.69,0.87);
#28429=FILL_AREA_STYLE_COLOUR('',#28428);
#28430=FILL_AREA_STYLE('',(#28429));
#28431=SURFACE_STYLE_FILL_AREA(#28430);
#28432=SURFACE_SIDE_STYLE('',(#28431));
#28433=SURFACE_STYLE_USAGE(.BOTH.,#28432);
#28434=PRESENTATION_STYLE_ASSIGNMENT((#28433));
ENDSEC;
END-ISO-10303-21;
